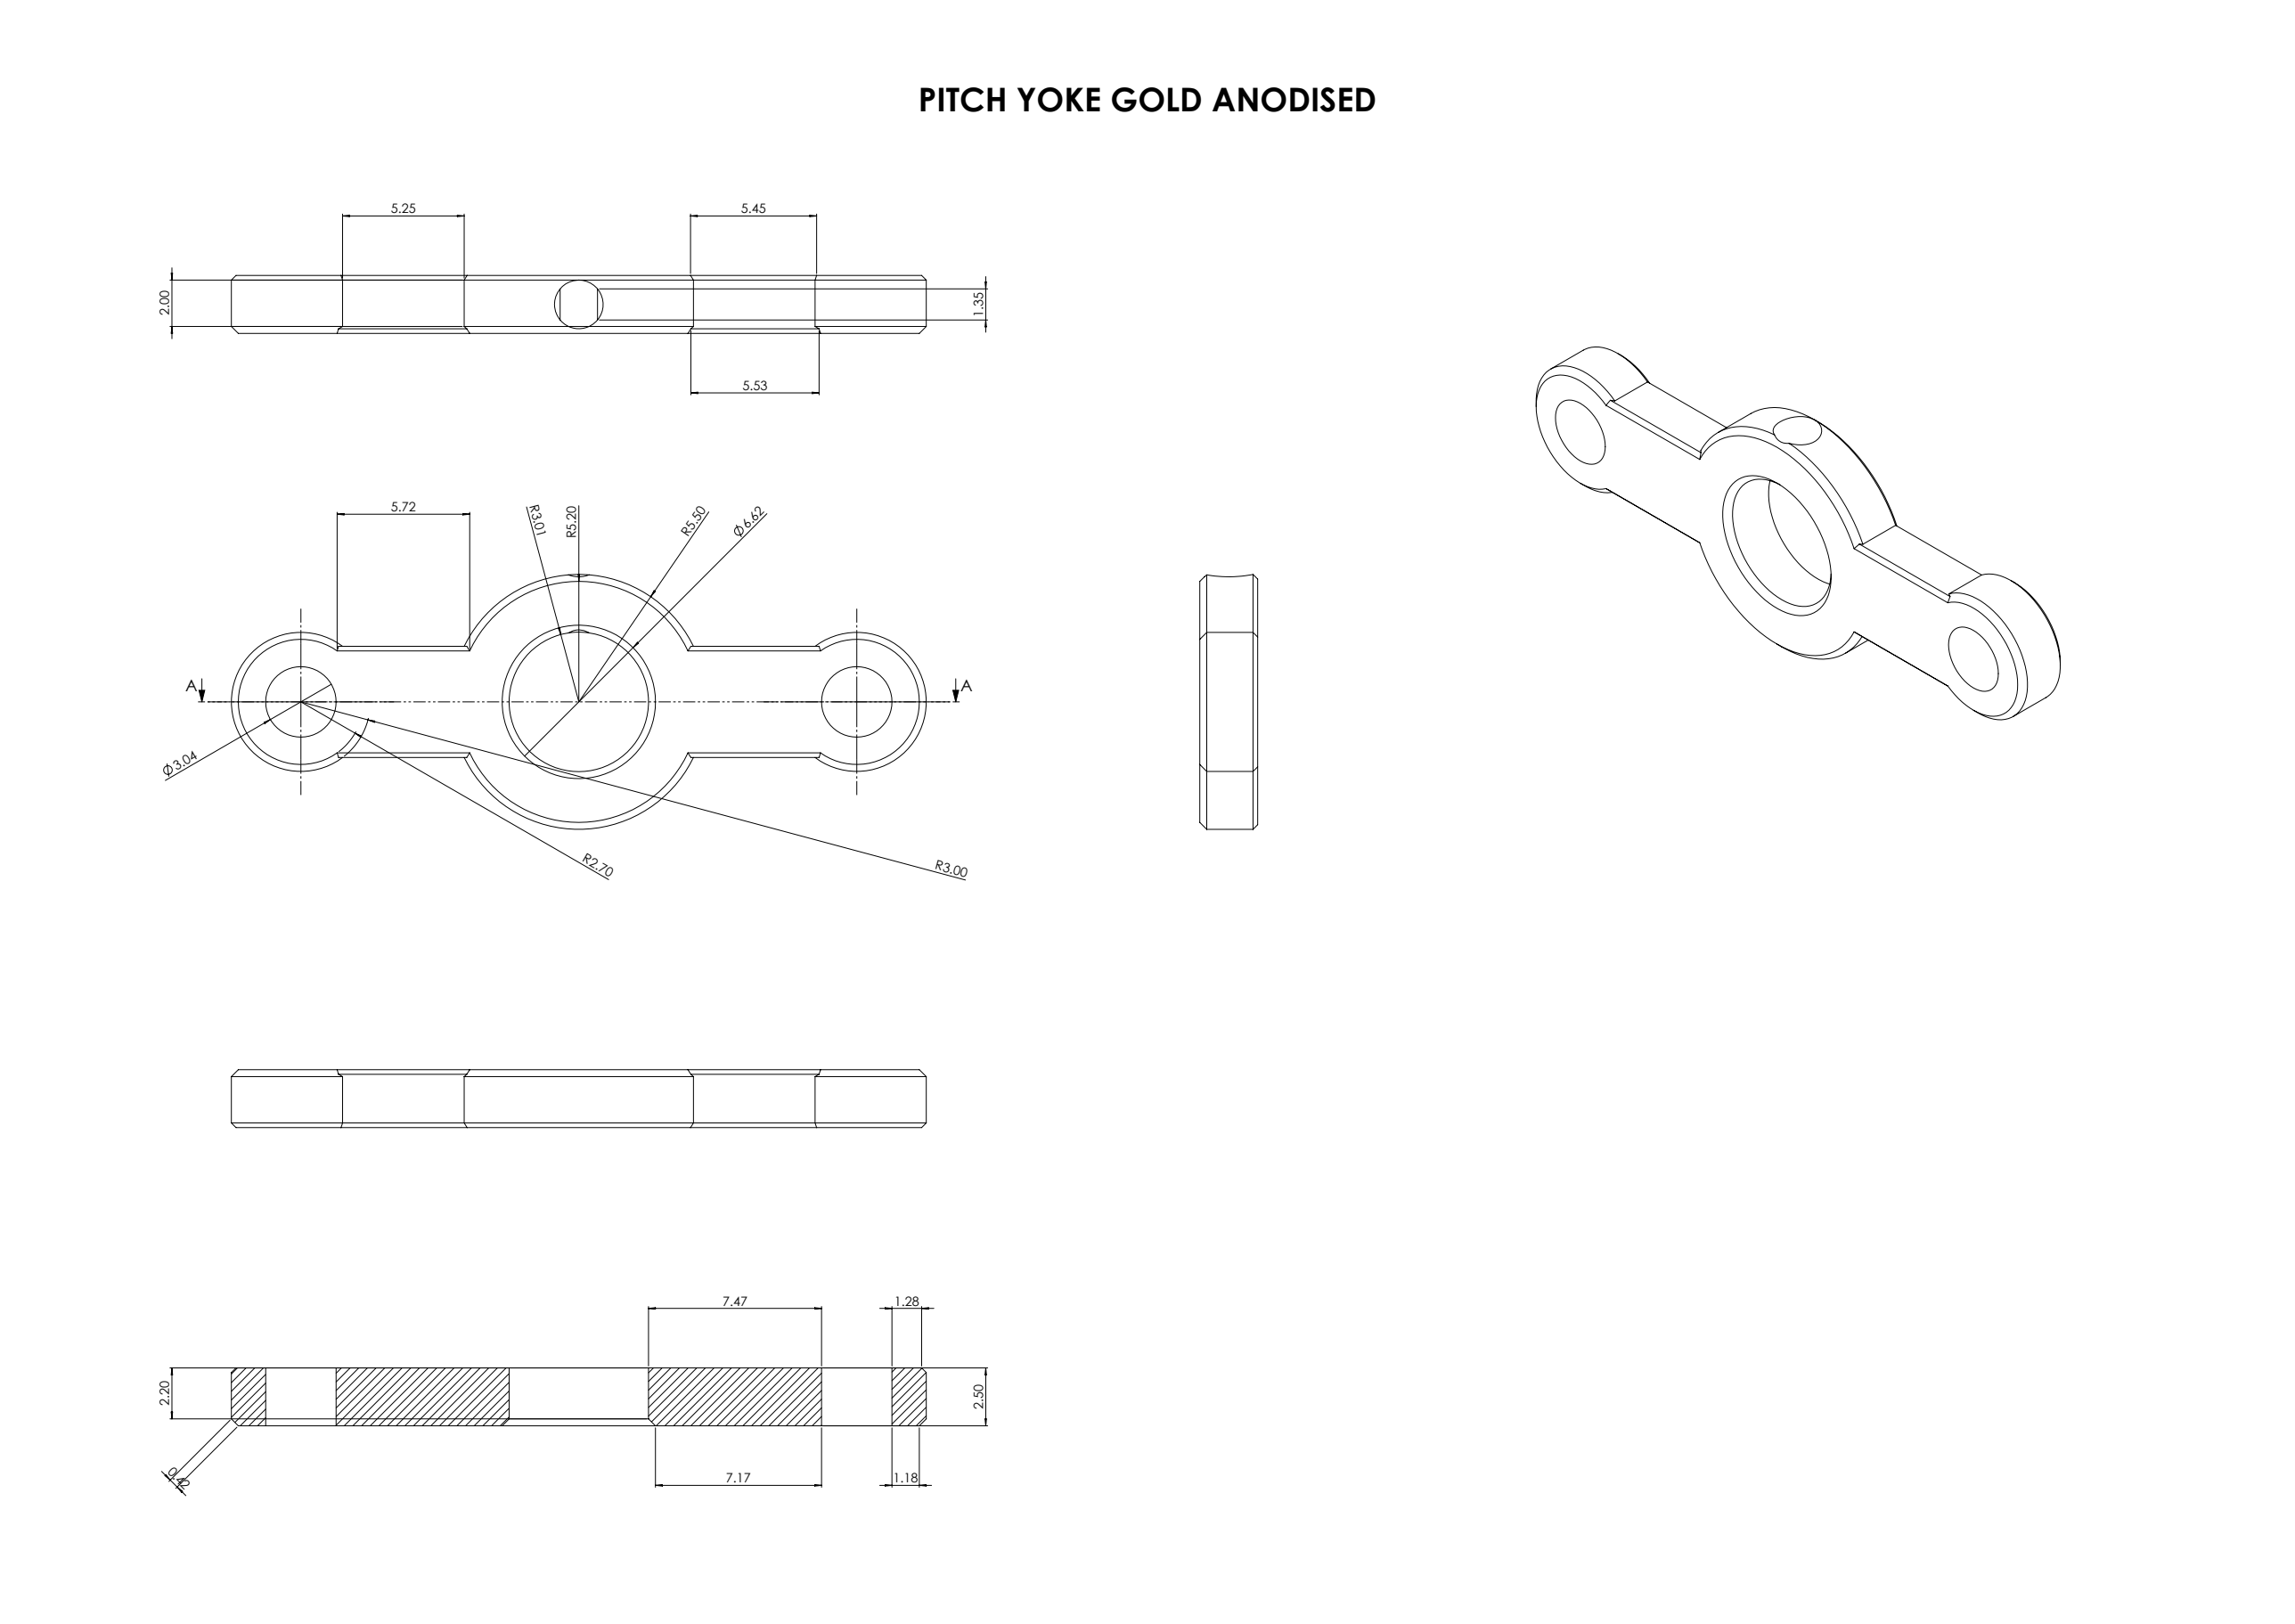
ISO-10303-21;
HEADER;
/* Generated by software containing ST-Developer
 * from STEP Tools, Inc. (www.steptools.com) 
 */

FILE_DESCRIPTION(
/* description */ (''),
/* implementation_level */ '2;1');

FILE_NAME(
/* name */ '05_Pitch_Yoke_Gold_Anodised.step',
/* time_stamp */ '2026-10-25T01:35:35-07:00',
/* author */ (''),
/* organization */ (''),
/* preprocessor_version */ 'ST-DEVELOPER v20.2',
/* originating_system */ 'Autodesk Translation Framework v15.15.0.0',
/* authorisation */ '');

FILE_SCHEMA (('AUTOMOTIVE_DESIGN { 1 0 10303 214 3 1 1 }'));
ENDSEC;

DATA;
#10=MECHANICAL_DESIGN_GEOMETRIC_PRESENTATION_REPRESENTATION('',(#264),#11430);
#86=B_SPLINE_CURVE_WITH_KNOTS('',3,(#6723,#6724,#6725,#6726),
 .UNSPECIFIED.,.F.,.F.,(4,4),(-0.0309968818258504,0.),.UNSPECIFIED.);
#87=B_SPLINE_CURVE_WITH_KNOTS('',3,(#6727,#6728,#6729,#6730),
 .UNSPECIFIED.,.F.,.F.,(4,4),(-0.0290771795561931,0.),.UNSPECIFIED.);
#88=B_SPLINE_CURVE_WITH_KNOTS('',3,(#6734,#6735,#6736,#6737),
 .UNSPECIFIED.,.F.,.F.,(4,4),(-0.0309968818257846,0.),.UNSPECIFIED.);
#89=B_SPLINE_CURVE_WITH_KNOTS('',3,(#6742,#6743,#6744,#6745),
 .UNSPECIFIED.,.F.,.F.,(4,4),(-0.0290773085804053,0.),.UNSPECIFIED.);
#90=B_SPLINE_CURVE_WITH_KNOTS('',3,(#6748,#6749,#6750,#6751),
 .UNSPECIFIED.,.F.,.F.,(4,4),(-0.0290771795561931,0.),.UNSPECIFIED.);
#91=B_SPLINE_CURVE_WITH_KNOTS('',3,(#6757,#6758,#6759,#6760),
 .UNSPECIFIED.,.F.,.F.,(4,4),(-0.0309968818258147,0.),.UNSPECIFIED.);
#92=B_SPLINE_CURVE_WITH_KNOTS('',3,(#6767,#6768,#6769,#6770),
 .UNSPECIFIED.,.F.,.F.,(4,4),(-0.030996881825835,0.),.UNSPECIFIED.);
#93=B_SPLINE_CURVE_WITH_KNOTS('',3,(#6774,#6775,#6776,#6777),
 .UNSPECIFIED.,.F.,.F.,(4,4),(-0.0290771795558996,0.),.UNSPECIFIED.);
#94=B_SPLINE_CURVE_WITH_KNOTS('',3,(#6787,#6788,#6789,#6790,#6791,#6792,
#6793,#6794,#6795,#6796,#6797,#6798,#6799,#6800,#6801,#6802,#6803),
 .UNSPECIFIED.,.F.,.F.,(4,2,2,2,3,2,2,4),(0.475883554626383,0.515539598201686,
0.555195641776989,0.594853523972749,0.63451140616851,0.674169288364271,
0.713827170560032,0.748840077704135),.UNSPECIFIED.);
#95=B_SPLINE_CURVE_WITH_KNOTS('',3,(#6818,#6819,#6820,#6821,#6822,#6823,
#6824,#6825,#6826,#6827),.UNSPECIFIED.,.F.,.F.,(4,2,2,2,4),(0.119476318069872,
0.130197921487587,0.164602551565189,0.199007181642792,0.209728785060507),
 .UNSPECIFIED.);
#96=B_SPLINE_CURVE_WITH_KNOTS('',3,(#6832,#6833,#6834,#6835,#6836,#6837,
#6838,#6839),.UNSPECIFIED.,.F.,.F.,(4,2,2,4),(0.20292703154863,0.237939938692733,
0.277597820888494,0.317255703084255),.UNSPECIFIED.);
#97=B_SPLINE_CURVE_WITH_KNOTS('',3,(#6840,#6841,#6842,#6843,#6844,#6845,
#6846,#6847,#6848,#6849),.UNSPECIFIED.,.F.,.F.,(4,2,2,2,4),(0.317255703084255,
0.356913585280016,0.396571467475777,0.43622751105108,0.475883554626383),
 .UNSPECIFIED.);
#98=B_SPLINE_CURVE_WITH_KNOTS('',3,(#6856,#6857,#6858,#6859,#6860,#6861,
#6862,#6863,#6864,#6865,#6866,#6867,#6868,#6869),.UNSPECIFIED.,.F.,.F.,
(4,2,2,2,2,2,4),(0.389725630667101,0.399201782687169,0.439108489087217,
0.479015195487264,0.518921901887312,0.55882860828736,0.568304760307428),
 .UNSPECIFIED.);
#99=B_SPLINE_CURVE_WITH_KNOTS('',3,(#6873,#6874,#6875,#6876,#6877,#6878),
 .UNSPECIFIED.,.F.,.F.,(4,2,4),(0.204141306797506,0.239485144629183,0.248961296649252),
 .UNSPECIFIED.);
#100=B_SPLINE_CURVE_WITH_KNOTS('',3,(#6880,#6881,#6882,#6883,#6884,#6885,
#6886,#6887,#6888,#6889),.UNSPECIFIED.,.F.,.F.,(4,2,2,2,4),(0.238592722720123,
0.259879734519813,0.28491657542964,0.309953416339467,0.331240428139157),
 .UNSPECIFIED.);
#101=B_SPLINE_CURVE_WITH_KNOTS('',3,(#6891,#6892,#6893,#6894,#6895,#6896),
 .UNSPECIFIED.,.F.,.F.,(4,2,4),(0.0703821670089247,0.079858319028993,0.115202156860671),
 .UNSPECIFIED.);
#220=(
BOUNDED_CURVE()
B_SPLINE_CURVE(2,(#6614,#6615,#6616),.UNSPECIFIED.,.F.,.F.)
B_SPLINE_CURVE_WITH_KNOTS((3,3),(0.,0.0309504086115576),.UNSPECIFIED.)
CURVE()
GEOMETRIC_REPRESENTATION_ITEM()
RATIONAL_B_SPLINE_CURVE((1.,1.,1.))
REPRESENTATION_ITEM('')
);
#221=(
BOUNDED_CURVE()
B_SPLINE_CURVE(2,(#6620,#6621,#6622),.UNSPECIFIED.,.F.,.F.)
B_SPLINE_CURVE_WITH_KNOTS((3,3),(0.,0.0289695421536074),.UNSPECIFIED.)
CURVE()
GEOMETRIC_REPRESENTATION_ITEM()
RATIONAL_B_SPLINE_CURVE((1.,1.,1.))
REPRESENTATION_ITEM('')
);
#222=(
BOUNDED_CURVE()
B_SPLINE_CURVE(2,(#6626,#6627,#6628),.UNSPECIFIED.,.F.,.F.)
B_SPLINE_CURVE_WITH_KNOTS((3,3),(0.0303639456287982,0.0450225821689597),
 .UNSPECIFIED.)
CURVE()
GEOMETRIC_REPRESENTATION_ITEM()
RATIONAL_B_SPLINE_CURVE((1.00021631089164,1.00016036906093,1.))
REPRESENTATION_ITEM('')
);
#223=(
BOUNDED_CURVE()
B_SPLINE_CURVE(2,(#6635,#6636,#6637),.UNSPECIFIED.,.F.,.F.)
B_SPLINE_CURVE_WITH_KNOTS((3,3),(0.,0.0187833832018332),.UNSPECIFIED.)
CURVE()
GEOMETRIC_REPRESENTATION_ITEM()
RATIONAL_B_SPLINE_CURVE((1.,1.0014465102333,1.00204161237231))
REPRESENTATION_ITEM('')
);
#224=(
BOUNDED_CURVE()
B_SPLINE_CURVE(2,(#6641,#6642,#6643),.UNSPECIFIED.,.F.,.F.)
B_SPLINE_CURVE_WITH_KNOTS((3,3),(0.,0.0289695421536071),.UNSPECIFIED.)
CURVE()
GEOMETRIC_REPRESENTATION_ITEM()
RATIONAL_B_SPLINE_CURVE((1.,1.,1.))
REPRESENTATION_ITEM('')
);
#225=(
BOUNDED_CURVE()
B_SPLINE_CURVE(2,(#6647,#6648,#6649),.UNSPECIFIED.,.F.,.F.)
B_SPLINE_CURVE_WITH_KNOTS((3,3),(0.,0.0309504086115573),.UNSPECIFIED.)
CURVE()
GEOMETRIC_REPRESENTATION_ITEM()
RATIONAL_B_SPLINE_CURVE((1.,1.,1.))
REPRESENTATION_ITEM('')
);
#226=(
BOUNDED_CURVE()
B_SPLINE_CURVE(2,(#6653,#6654,#6655),.UNSPECIFIED.,.F.,.F.)
B_SPLINE_CURVE_WITH_KNOTS((3,3),(0.0450411357331602,0.0638245189349933),
 .UNSPECIFIED.)
CURVE()
GEOMETRIC_REPRESENTATION_ITEM()
RATIONAL_B_SPLINE_CURVE((1.00204161237231,1.0014465102333,1.))
REPRESENTATION_ITEM('')
);
#227=(
BOUNDED_CURVE()
B_SPLINE_CURVE(2,(#6662,#6663,#6664),.UNSPECIFIED.,.F.,.F.)
B_SPLINE_CURVE_WITH_KNOTS((3,3),(0.,0.0146586365398684),.UNSPECIFIED.)
CURVE()
GEOMETRIC_REPRESENTATION_ITEM()
RATIONAL_B_SPLINE_CURVE((1.,1.00016036906092,1.00021631089164))
REPRESENTATION_ITEM('')
);
#228=(
BOUNDED_CURVE()
B_SPLINE_CURVE(2,(#6668,#6669,#6670),.UNSPECIFIED.,.F.,.F.)
B_SPLINE_CURVE_WITH_KNOTS((3,3),(0.,0.0309504086115573),.UNSPECIFIED.)
CURVE()
GEOMETRIC_REPRESENTATION_ITEM()
RATIONAL_B_SPLINE_CURVE((1.,1.,1.))
REPRESENTATION_ITEM('')
);
#229=(
BOUNDED_CURVE()
B_SPLINE_CURVE(2,(#6674,#6675,#6676),.UNSPECIFIED.,.F.,.F.)
B_SPLINE_CURVE_WITH_KNOTS((3,3),(0.,0.0289695421536071),.UNSPECIFIED.)
CURVE()
GEOMETRIC_REPRESENTATION_ITEM()
RATIONAL_B_SPLINE_CURVE((1.,1.,1.))
REPRESENTATION_ITEM('')
);
#230=(
BOUNDED_CURVE()
B_SPLINE_CURVE(2,(#6680,#6681,#6682),.UNSPECIFIED.,.F.,.F.)
B_SPLINE_CURVE_WITH_KNOTS((3,3),(0.0303678686581102,0.0450284286877096),
 .UNSPECIFIED.)
CURVE()
GEOMETRIC_REPRESENTATION_ITEM()
RATIONAL_B_SPLINE_CURVE((1.00021903389143,1.00016374915722,1.00000403669809))
REPRESENTATION_ITEM('')
);
#231=(
BOUNDED_CURVE()
B_SPLINE_CURVE(2,(#6689,#6690,#6691),.UNSPECIFIED.,.F.,.F.)
B_SPLINE_CURVE_WITH_KNOTS((3,3),(0.,0.0187833832018332),.UNSPECIFIED.)
CURVE()
GEOMETRIC_REPRESENTATION_ITEM()
RATIONAL_B_SPLINE_CURVE((1.,1.0014465102333,1.00204161237231))
REPRESENTATION_ITEM('')
);
#232=(
BOUNDED_CURVE()
B_SPLINE_CURVE(2,(#6695,#6696,#6697),.UNSPECIFIED.,.F.,.F.)
B_SPLINE_CURVE_WITH_KNOTS((3,3),(0.,0.0289695421536071),.UNSPECIFIED.)
CURVE()
GEOMETRIC_REPRESENTATION_ITEM()
RATIONAL_B_SPLINE_CURVE((1.,1.,1.))
REPRESENTATION_ITEM('')
);
#233=(
BOUNDED_CURVE()
B_SPLINE_CURVE(2,(#6701,#6702,#6703),.UNSPECIFIED.,.F.,.F.)
B_SPLINE_CURVE_WITH_KNOTS((3,3),(0.,0.0309504086115573),.UNSPECIFIED.)
CURVE()
GEOMETRIC_REPRESENTATION_ITEM()
RATIONAL_B_SPLINE_CURVE((1.,1.,1.))
REPRESENTATION_ITEM('')
);
#234=(
BOUNDED_CURVE()
B_SPLINE_CURVE(2,(#6707,#6708,#6709),.UNSPECIFIED.,.F.,.F.)
B_SPLINE_CURVE_WITH_KNOTS((3,3),(0.0450411357331602,0.0638245189349933),
 .UNSPECIFIED.)
CURVE()
GEOMETRIC_REPRESENTATION_ITEM()
RATIONAL_B_SPLINE_CURVE((1.00204161237231,1.0014465102333,1.))
REPRESENTATION_ITEM('')
);
#235=(
BOUNDED_CURVE()
B_SPLINE_CURVE(2,(#6716,#6717,#6718),.UNSPECIFIED.,.F.,.F.)
B_SPLINE_CURVE_WITH_KNOTS((3,3),(0.,0.014658636844145),.UNSPECIFIED.)
CURVE()
GEOMETRIC_REPRESENTATION_ITEM()
RATIONAL_B_SPLINE_CURVE((1.,1.00016036906825,1.00021631090007))
REPRESENTATION_ITEM('')
);
#240=SHAPE_REPRESENTATION_RELATIONSHIP('SRR','None',#11483,#252);
#252=ADVANCED_BREP_SHAPE_REPRESENTATION('',(#276),#11422);
#264=STYLED_ITEM('',(#11623),#276);
#276=MANIFOLD_SOLID_BREP('Body1',#4465);
#300=FACE_BOUND('',#901,.T.);
#301=FACE_BOUND('',#902,.T.);
#302=FACE_BOUND('',#903,.T.);
#303=FACE_BOUND('',#912,.T.);
#304=FACE_BOUND('',#913,.T.);
#305=FACE_BOUND('',#914,.T.);
#353=PLANE('',#4743);
#354=PLANE('',#4744);
#355=PLANE('',#4745);
#356=PLANE('',#4746);
#357=PLANE('',#4747);
#358=PLANE('',#4748);
#359=PLANE('',#4749);
#360=PLANE('',#4750);
#361=PLANE('',#4751);
#362=PLANE('',#4758);
#363=PLANE('',#4759);
#364=PLANE('',#4764);
#365=PLANE('',#4776);
#366=PLANE('',#4798);
#367=PLANE('',#4801);
#368=PLANE('',#4802);
#447=CYLINDRICAL_SURFACE('',#4768,3.);
#448=CYLINDRICAL_SURFACE('',#4770,5.5);
#449=CYLINDRICAL_SURFACE('',#4772,5.5);
#450=CYLINDRICAL_SURFACE('',#4774,3.);
#451=CYLINDRICAL_SURFACE('',#4785,5.5);
#452=CYLINDRICAL_SURFACE('',#4786,1.05);
#453=CYLINDRICAL_SURFACE('',#4803,1.52);
#454=CYLINDRICAL_SURFACE('',#4804,1.52);
#455=CYLINDRICAL_SURFACE('',#4805,3.01);
#596=FACE_OUTER_BOUND('',#880,.T.);
#597=FACE_OUTER_BOUND('',#881,.T.);
#598=FACE_OUTER_BOUND('',#882,.T.);
#599=FACE_OUTER_BOUND('',#883,.T.);
#600=FACE_OUTER_BOUND('',#884,.T.);
#601=FACE_OUTER_BOUND('',#885,.T.);
#602=FACE_OUTER_BOUND('',#886,.T.);
#603=FACE_OUTER_BOUND('',#887,.T.);
#604=FACE_OUTER_BOUND('',#888,.T.);
#605=FACE_OUTER_BOUND('',#889,.T.);
#606=FACE_OUTER_BOUND('',#890,.T.);
#607=FACE_OUTER_BOUND('',#891,.T.);
#608=FACE_OUTER_BOUND('',#892,.T.);
#609=FACE_OUTER_BOUND('',#893,.T.);
#610=FACE_OUTER_BOUND('',#894,.T.);
#611=FACE_OUTER_BOUND('',#895,.T.);
#612=FACE_OUTER_BOUND('',#896,.T.);
#613=FACE_OUTER_BOUND('',#897,.T.);
#614=FACE_OUTER_BOUND('',#898,.T.);
#615=FACE_OUTER_BOUND('',#899,.T.);
#616=FACE_OUTER_BOUND('',#900,.T.);
#617=FACE_OUTER_BOUND('',#904,.T.);
#618=FACE_OUTER_BOUND('',#905,.T.);
#619=FACE_OUTER_BOUND('',#906,.T.);
#620=FACE_OUTER_BOUND('',#907,.T.);
#621=FACE_OUTER_BOUND('',#908,.T.);
#622=FACE_OUTER_BOUND('',#909,.T.);
#623=FACE_OUTER_BOUND('',#910,.T.);
#624=FACE_OUTER_BOUND('',#911,.T.);
#625=FACE_OUTER_BOUND('',#915,.T.);
#626=FACE_OUTER_BOUND('',#916,.T.);
#627=FACE_OUTER_BOUND('',#917,.T.);
#628=FACE_OUTER_BOUND('',#918,.T.);
#629=FACE_OUTER_BOUND('',#919,.T.);
#880=EDGE_LOOP('',(#3147,#3148,#3149,#3150));
#881=EDGE_LOOP('',(#3151,#3152,#3153,#3154,#3155,#3156));
#882=EDGE_LOOP('',(#3157,#3158,#3159,#3160));
#883=EDGE_LOOP('',(#3161,#3162,#3163,#3164,#3165,#3166));
#884=EDGE_LOOP('',(#3167,#3168,#3169,#3170));
#885=EDGE_LOOP('',(#3171,#3172,#3173,#3174,#3175,#3176));
#886=EDGE_LOOP('',(#3177,#3178,#3179,#3180));
#887=EDGE_LOOP('',(#3181,#3182,#3183,#3184,#3185,#3186));
#888=EDGE_LOOP('',(#3187,#3188,#3189,#3190));
#889=EDGE_LOOP('',(#3191,#3192,#3193,#3194));
#890=EDGE_LOOP('',(#3195,#3196,#3197,#3198));
#891=EDGE_LOOP('',(#3199,#3200,#3201,#3202));
#892=EDGE_LOOP('',(#3203,#3204,#3205,#3206));
#893=EDGE_LOOP('',(#3207,#3208,#3209,#3210,#3211));
#894=EDGE_LOOP('',(#3212,#3213,#3214,#3215));
#895=EDGE_LOOP('',(#3216,#3217,#3218,#3219));
#896=EDGE_LOOP('',(#3220,#3221,#3222,#3223));
#897=EDGE_LOOP('',(#3224,#3225,#3226,#3227));
#898=EDGE_LOOP('',(#3228,#3229,#3230,#3231));
#899=EDGE_LOOP('',(#3232,#3233,#3234,#3235));
#900=EDGE_LOOP('',(#3236,#3237,#3238,#3239,#3240,#3241,#3242,#3243));
#901=EDGE_LOOP('',(#3244));
#902=EDGE_LOOP('',(#3245));
#903=EDGE_LOOP('',(#3246));
#904=EDGE_LOOP('',(#3247,#3248,#3249,#3250,#3251,#3252));
#905=EDGE_LOOP('',(#3253,#3254,#3255,#3256,#3257,#3258,#3259,#3260));
#906=EDGE_LOOP('',(#3261,#3262,#3263,#3264,#3265));
#907=EDGE_LOOP('',(#3266,#3267,#3268,#3269,#3270,#3271,#3272,#3273,#3274,
#3275,#3276,#3277,#3278));
#908=EDGE_LOOP('',(#3279,#3280,#3281,#3282,#3283,#3284));
#909=EDGE_LOOP('',(#3285,#3286,#3287,#3288,#3289,#3290));
#910=EDGE_LOOP('',(#3291,#3292,#3293,#3294,#3295,#3296));
#911=EDGE_LOOP('',(#3297,#3298,#3299,#3300,#3301,#3302,#3303,#3304));
#912=EDGE_LOOP('',(#3305));
#913=EDGE_LOOP('',(#3306));
#914=EDGE_LOOP('',(#3307));
#915=EDGE_LOOP('',(#3308,#3309,#3310));
#916=EDGE_LOOP('',(#3311,#3312));
#917=EDGE_LOOP('',(#3313,#3314,#3315,#3316));
#918=EDGE_LOOP('',(#3317,#3318,#3319,#3320));
#919=EDGE_LOOP('',(#3321,#3322,#3323,#3324,#3325,#3326,#3327,#3328,#3329,
#3330));
#1171=LINE('',#6618,#1461);
#1172=LINE('',#6623,#1462);
#1173=LINE('',#6630,#1463);
#1174=LINE('',#6632,#1464);
#1175=LINE('',#6634,#1465);
#1176=LINE('',#6645,#1466);
#1177=LINE('',#6650,#1467);
#1178=LINE('',#6657,#1468);
#1179=LINE('',#6659,#1469);
#1180=LINE('',#6661,#1470);
#1181=LINE('',#6672,#1471);
#1182=LINE('',#6677,#1472);
#1183=LINE('',#6684,#1473);
#1184=LINE('',#6686,#1474);
#1185=LINE('',#6688,#1475);
#1186=LINE('',#6699,#1476);
#1187=LINE('',#6704,#1477);
#1188=LINE('',#6711,#1478);
#1189=LINE('',#6713,#1479);
#1190=LINE('',#6715,#1480);
#1191=LINE('',#6722,#1481);
#1192=LINE('',#6753,#1482);
#1193=LINE('',#6756,#1483);
#1194=LINE('',#6773,#1484);
#1195=LINE('',#6852,#1485);
#1196=LINE('',#6906,#1486);
#1197=LINE('',#6915,#1487);
#1198=LINE('',#6917,#1488);
#1199=LINE('',#6919,#1489);
#1200=LINE('',#6921,#1490);
#1201=LINE('',#6923,#1491);
#1461=VECTOR('',#5429,10.);
#1462=VECTOR('',#5430,10.);
#1463=VECTOR('',#5433,10.);
#1464=VECTOR('',#5434,10.);
#1465=VECTOR('',#5435,10.);
#1466=VECTOR('',#5438,10.);
#1467=VECTOR('',#5439,10.);
#1468=VECTOR('',#5442,10.);
#1469=VECTOR('',#5443,10.);
#1470=VECTOR('',#5444,10.);
#1471=VECTOR('',#5447,10.);
#1472=VECTOR('',#5448,10.);
#1473=VECTOR('',#5451,10.);
#1474=VECTOR('',#5452,10.);
#1475=VECTOR('',#5453,10.);
#1476=VECTOR('',#5456,10.);
#1477=VECTOR('',#5457,10.);
#1478=VECTOR('',#5460,10.);
#1479=VECTOR('',#5461,10.);
#1480=VECTOR('',#5462,10.);
#1481=VECTOR('',#5465,10.);
#1482=VECTOR('',#5480,10.);
#1483=VECTOR('',#5483,10.);
#1484=VECTOR('',#5494,10.);
#1485=VECTOR('',#5539,1.05);
#1486=VECTOR('',#5558,3.16);
#1487=VECTOR('',#5571,10.);
#1488=VECTOR('',#5574,10.);
#1489=VECTOR('',#5577,1.52);
#1490=VECTOR('',#5580,1.52);
#1491=VECTOR('',#5583,3.01);
#1742=CIRCLE('',#4753,5.3);
#1743=CIRCLE('',#4754,5.5);
#1744=CIRCLE('',#4756,3.);
#1745=CIRCLE('',#4757,2.8);
#1746=CIRCLE('',#4761,5.5);
#1747=CIRCLE('',#4762,5.5);
#1748=CIRCLE('',#4763,5.3);
#1749=CIRCLE('',#4766,3.);
#1750=CIRCLE('',#4767,2.8);
#1751=CIRCLE('',#4769,3.);
#1752=CIRCLE('',#4771,5.5);
#1753=CIRCLE('',#4773,5.5);
#1754=CIRCLE('',#4775,3.);
#1755=CIRCLE('',#4777,3.01);
#1756=CIRCLE('',#4778,1.52);
#1757=CIRCLE('',#4779,1.52);
#1758=CIRCLE('',#4781,2.7);
#1759=CIRCLE('',#4783,5.5);
#1760=CIRCLE('',#4784,5.2);
#1761=CIRCLE('',#4787,1.05);
#1762=CIRCLE('',#4788,1.05);
#1763=CIRCLE('',#4789,1.05);
#1764=CIRCLE('',#4791,2.7);
#1765=CIRCLE('',#4793,5.2);
#1766=CIRCLE('',#4795,3.31);
#1767=CIRCLE('',#4796,3.01);
#1768=CIRCLE('',#4797,3.01);
#1769=CIRCLE('',#4799,1.52);
#1770=CIRCLE('',#4800,1.52);
#1943=VERTEX_POINT('',#6612);
#1944=VERTEX_POINT('',#6613);
#1945=VERTEX_POINT('',#6617);
#1946=VERTEX_POINT('',#6619);
#1947=VERTEX_POINT('',#6625);
#1948=VERTEX_POINT('',#6629);
#1949=VERTEX_POINT('',#6631);
#1950=VERTEX_POINT('',#6633);
#1951=VERTEX_POINT('',#6639);
#1952=VERTEX_POINT('',#6640);
#1953=VERTEX_POINT('',#6644);
#1954=VERTEX_POINT('',#6646);
#1955=VERTEX_POINT('',#6652);
#1956=VERTEX_POINT('',#6656);
#1957=VERTEX_POINT('',#6658);
#1958=VERTEX_POINT('',#6660);
#1959=VERTEX_POINT('',#6666);
#1960=VERTEX_POINT('',#6667);
#1961=VERTEX_POINT('',#6671);
#1962=VERTEX_POINT('',#6673);
#1963=VERTEX_POINT('',#6679);
#1964=VERTEX_POINT('',#6683);
#1965=VERTEX_POINT('',#6685);
#1966=VERTEX_POINT('',#6687);
#1967=VERTEX_POINT('',#6693);
#1968=VERTEX_POINT('',#6694);
#1969=VERTEX_POINT('',#6698);
#1970=VERTEX_POINT('',#6700);
#1971=VERTEX_POINT('',#6706);
#1972=VERTEX_POINT('',#6710);
#1973=VERTEX_POINT('',#6712);
#1974=VERTEX_POINT('',#6714);
#1975=VERTEX_POINT('',#6720);
#1976=VERTEX_POINT('',#6721);
#1977=VERTEX_POINT('',#6732);
#1978=VERTEX_POINT('',#6741);
#1979=VERTEX_POINT('',#6746);
#1980=VERTEX_POINT('',#6755);
#1981=VERTEX_POINT('',#6762);
#1982=VERTEX_POINT('',#6765);
#1983=VERTEX_POINT('',#6772);
#1984=VERTEX_POINT('',#6786);
#1985=VERTEX_POINT('',#6808);
#1986=VERTEX_POINT('',#6810);
#1987=VERTEX_POINT('',#6812);
#1988=VERTEX_POINT('',#6817);
#1989=VERTEX_POINT('',#6831);
#1990=VERTEX_POINT('',#6851);
#1991=VERTEX_POINT('',#6853);
#1992=VERTEX_POINT('',#6855);
#1993=VERTEX_POINT('',#6870);
#1994=VERTEX_POINT('',#6872);
#1995=VERTEX_POINT('',#6879);
#1996=VERTEX_POINT('',#6890);
#1997=VERTEX_POINT('',#6903);
#1998=VERTEX_POINT('',#6905);
#1999=VERTEX_POINT('',#6910);
#2000=VERTEX_POINT('',#6912);
#2391=EDGE_CURVE('',#1943,#1944,#220,.F.);
#2392=EDGE_CURVE('',#1944,#1945,#1171,.T.);
#2393=EDGE_CURVE('',#1945,#1946,#221,.F.);
#2394=EDGE_CURVE('',#1946,#1943,#1172,.T.);
#2395=EDGE_CURVE('',#1947,#1944,#222,.F.);
#2396=EDGE_CURVE('',#1948,#1947,#1173,.T.);
#2397=EDGE_CURVE('',#1949,#1948,#1174,.T.);
#2398=EDGE_CURVE('',#1949,#1950,#1175,.T.);
#2399=EDGE_CURVE('',#1945,#1950,#223,.F.);
#2400=EDGE_CURVE('',#1951,#1952,#224,.F.);
#2401=EDGE_CURVE('',#1952,#1953,#1176,.T.);
#2402=EDGE_CURVE('',#1953,#1954,#225,.F.);
#2403=EDGE_CURVE('',#1954,#1951,#1177,.T.);
#2404=EDGE_CURVE('',#1955,#1952,#226,.F.);
#2405=EDGE_CURVE('',#1956,#1955,#1178,.T.);
#2406=EDGE_CURVE('',#1957,#1956,#1179,.T.);
#2407=EDGE_CURVE('',#1957,#1958,#1180,.T.);
#2408=EDGE_CURVE('',#1953,#1958,#227,.F.);
#2409=EDGE_CURVE('',#1959,#1960,#228,.F.);
#2410=EDGE_CURVE('',#1960,#1961,#1181,.T.);
#2411=EDGE_CURVE('',#1961,#1962,#229,.F.);
#2412=EDGE_CURVE('',#1962,#1959,#1182,.T.);
#2413=EDGE_CURVE('',#1963,#1960,#230,.F.);
#2414=EDGE_CURVE('',#1964,#1963,#1183,.T.);
#2415=EDGE_CURVE('',#1965,#1964,#1184,.T.);
#2416=EDGE_CURVE('',#1965,#1966,#1185,.T.);
#2417=EDGE_CURVE('',#1961,#1966,#231,.F.);
#2418=EDGE_CURVE('',#1967,#1968,#232,.F.);
#2419=EDGE_CURVE('',#1968,#1969,#1186,.T.);
#2420=EDGE_CURVE('',#1969,#1970,#233,.F.);
#2421=EDGE_CURVE('',#1970,#1967,#1187,.T.);
#2422=EDGE_CURVE('',#1971,#1968,#234,.F.);
#2423=EDGE_CURVE('',#1972,#1971,#1188,.T.);
#2424=EDGE_CURVE('',#1973,#1972,#1189,.T.);
#2425=EDGE_CURVE('',#1973,#1974,#1190,.T.);
#2426=EDGE_CURVE('',#1969,#1974,#235,.F.);
#2427=EDGE_CURVE('',#1975,#1976,#1191,.T.);
#2428=EDGE_CURVE('',#1976,#1957,#86,.T.);
#2429=EDGE_CURVE('',#1975,#1956,#87,.T.);
#2430=EDGE_CURVE('',#1976,#1977,#1742,.T.);
#2431=EDGE_CURVE('',#1977,#1948,#88,.T.);
#2432=EDGE_CURVE('',#1948,#1957,#1743,.T.);
#2433=EDGE_CURVE('',#1972,#1949,#1744,.T.);
#2434=EDGE_CURVE('',#1949,#1978,#89,.T.);
#2435=EDGE_CURVE('',#1978,#1979,#1745,.T.);
#2436=EDGE_CURVE('',#1979,#1972,#90,.T.);
#2437=EDGE_CURVE('',#1977,#1978,#1192,.T.);
#2438=EDGE_CURVE('',#1979,#1980,#1193,.T.);
#2439=EDGE_CURVE('',#1980,#1973,#91,.T.);
#2440=EDGE_CURVE('',#1964,#1981,#1746,.T.);
#2441=EDGE_CURVE('',#1981,#1973,#1747,.T.);
#2442=EDGE_CURVE('',#1980,#1982,#1748,.T.);
#2443=EDGE_CURVE('',#1982,#1964,#92,.T.);
#2444=EDGE_CURVE('',#1982,#1983,#1194,.T.);
#2445=EDGE_CURVE('',#1983,#1965,#93,.T.);
#2446=EDGE_CURVE('',#1956,#1965,#1749,.T.);
#2447=EDGE_CURVE('',#1983,#1975,#1750,.T.);
#2448=EDGE_CURVE('',#1966,#1955,#1751,.T.);
#2449=EDGE_CURVE('',#1958,#1947,#1752,.T.);
#2450=EDGE_CURVE('',#1981,#1984,#94,.T.);
#2451=EDGE_CURVE('',#1974,#1984,#1753,.T.);
#2452=EDGE_CURVE('',#1950,#1971,#1754,.T.);
#2453=EDGE_CURVE('',#1985,#1985,#1755,.T.);
#2454=EDGE_CURVE('',#1986,#1986,#1756,.T.);
#2455=EDGE_CURVE('',#1987,#1987,#1757,.T.);
#2456=EDGE_CURVE('',#1967,#1946,#1758,.T.);
#2457=EDGE_CURVE('',#1984,#1988,#95,.T.);
#2458=EDGE_CURVE('',#1988,#1963,#1759,.T.);
#2459=EDGE_CURVE('',#1959,#1970,#1760,.T.);
#2460=EDGE_CURVE('',#1988,#1989,#96,.T.);
#2461=EDGE_CURVE('',#1989,#1981,#97,.T.);
#2462=EDGE_CURVE('',#1989,#1990,#1195,.T.);
#2463=EDGE_CURVE('',#1990,#1991,#1761,.T.);
#2464=EDGE_CURVE('',#1992,#1991,#98,.T.);
#2465=EDGE_CURVE('',#1992,#1993,#1762,.T.);
#2466=EDGE_CURVE('',#1994,#1993,#99,.T.);
#2467=EDGE_CURVE('',#1995,#1994,#100,.T.);
#2468=EDGE_CURVE('',#1996,#1995,#101,.T.);
#2469=EDGE_CURVE('',#1996,#1990,#1763,.T.);
#2470=EDGE_CURVE('',#1951,#1962,#1764,.T.);
#2471=EDGE_CURVE('',#1943,#1954,#1765,.T.);
#2472=EDGE_CURVE('',#1997,#1997,#1766,.T.);
#2473=EDGE_CURVE('',#1997,#1998,#1196,.T.);
#2474=EDGE_CURVE('',#1998,#1995,#1767,.T.);
#2475=EDGE_CURVE('',#1994,#1998,#1768,.T.);
#2476=EDGE_CURVE('',#1999,#1999,#1769,.T.);
#2477=EDGE_CURVE('',#2000,#2000,#1770,.T.);
#2478=EDGE_CURVE('',#1991,#1996,#1197,.T.);
#2479=EDGE_CURVE('',#1993,#1992,#1198,.T.);
#2480=EDGE_CURVE('',#2000,#1987,#1199,.T.);
#2481=EDGE_CURVE('',#1999,#1986,#1200,.T.);
#2482=EDGE_CURVE('',#1998,#1985,#1201,.T.);
#3147=ORIENTED_EDGE('',*,*,#2391,.T.);
#3148=ORIENTED_EDGE('',*,*,#2392,.T.);
#3149=ORIENTED_EDGE('',*,*,#2393,.T.);
#3150=ORIENTED_EDGE('',*,*,#2394,.T.);
#3151=ORIENTED_EDGE('',*,*,#2392,.F.);
#3152=ORIENTED_EDGE('',*,*,#2395,.F.);
#3153=ORIENTED_EDGE('',*,*,#2396,.F.);
#3154=ORIENTED_EDGE('',*,*,#2397,.F.);
#3155=ORIENTED_EDGE('',*,*,#2398,.T.);
#3156=ORIENTED_EDGE('',*,*,#2399,.F.);
#3157=ORIENTED_EDGE('',*,*,#2400,.T.);
#3158=ORIENTED_EDGE('',*,*,#2401,.T.);
#3159=ORIENTED_EDGE('',*,*,#2402,.T.);
#3160=ORIENTED_EDGE('',*,*,#2403,.T.);
#3161=ORIENTED_EDGE('',*,*,#2401,.F.);
#3162=ORIENTED_EDGE('',*,*,#2404,.F.);
#3163=ORIENTED_EDGE('',*,*,#2405,.F.);
#3164=ORIENTED_EDGE('',*,*,#2406,.F.);
#3165=ORIENTED_EDGE('',*,*,#2407,.T.);
#3166=ORIENTED_EDGE('',*,*,#2408,.F.);
#3167=ORIENTED_EDGE('',*,*,#2409,.T.);
#3168=ORIENTED_EDGE('',*,*,#2410,.T.);
#3169=ORIENTED_EDGE('',*,*,#2411,.T.);
#3170=ORIENTED_EDGE('',*,*,#2412,.T.);
#3171=ORIENTED_EDGE('',*,*,#2410,.F.);
#3172=ORIENTED_EDGE('',*,*,#2413,.F.);
#3173=ORIENTED_EDGE('',*,*,#2414,.F.);
#3174=ORIENTED_EDGE('',*,*,#2415,.F.);
#3175=ORIENTED_EDGE('',*,*,#2416,.T.);
#3176=ORIENTED_EDGE('',*,*,#2417,.F.);
#3177=ORIENTED_EDGE('',*,*,#2418,.T.);
#3178=ORIENTED_EDGE('',*,*,#2419,.T.);
#3179=ORIENTED_EDGE('',*,*,#2420,.T.);
#3180=ORIENTED_EDGE('',*,*,#2421,.T.);
#3181=ORIENTED_EDGE('',*,*,#2419,.F.);
#3182=ORIENTED_EDGE('',*,*,#2422,.F.);
#3183=ORIENTED_EDGE('',*,*,#2423,.F.);
#3184=ORIENTED_EDGE('',*,*,#2424,.F.);
#3185=ORIENTED_EDGE('',*,*,#2425,.T.);
#3186=ORIENTED_EDGE('',*,*,#2426,.F.);
#3187=ORIENTED_EDGE('',*,*,#2427,.T.);
#3188=ORIENTED_EDGE('',*,*,#2428,.T.);
#3189=ORIENTED_EDGE('',*,*,#2406,.T.);
#3190=ORIENTED_EDGE('',*,*,#2429,.F.);
#3191=ORIENTED_EDGE('',*,*,#2430,.T.);
#3192=ORIENTED_EDGE('',*,*,#2431,.T.);
#3193=ORIENTED_EDGE('',*,*,#2432,.T.);
#3194=ORIENTED_EDGE('',*,*,#2428,.F.);
#3195=ORIENTED_EDGE('',*,*,#2433,.T.);
#3196=ORIENTED_EDGE('',*,*,#2434,.T.);
#3197=ORIENTED_EDGE('',*,*,#2435,.T.);
#3198=ORIENTED_EDGE('',*,*,#2436,.T.);
#3199=ORIENTED_EDGE('',*,*,#2437,.T.);
#3200=ORIENTED_EDGE('',*,*,#2434,.F.);
#3201=ORIENTED_EDGE('',*,*,#2397,.T.);
#3202=ORIENTED_EDGE('',*,*,#2431,.F.);
#3203=ORIENTED_EDGE('',*,*,#2424,.T.);
#3204=ORIENTED_EDGE('',*,*,#2436,.F.);
#3205=ORIENTED_EDGE('',*,*,#2438,.T.);
#3206=ORIENTED_EDGE('',*,*,#2439,.T.);
#3207=ORIENTED_EDGE('',*,*,#2440,.T.);
#3208=ORIENTED_EDGE('',*,*,#2441,.T.);
#3209=ORIENTED_EDGE('',*,*,#2439,.F.);
#3210=ORIENTED_EDGE('',*,*,#2442,.T.);
#3211=ORIENTED_EDGE('',*,*,#2443,.T.);
#3212=ORIENTED_EDGE('',*,*,#2415,.T.);
#3213=ORIENTED_EDGE('',*,*,#2443,.F.);
#3214=ORIENTED_EDGE('',*,*,#2444,.T.);
#3215=ORIENTED_EDGE('',*,*,#2445,.T.);
#3216=ORIENTED_EDGE('',*,*,#2446,.T.);
#3217=ORIENTED_EDGE('',*,*,#2445,.F.);
#3218=ORIENTED_EDGE('',*,*,#2447,.T.);
#3219=ORIENTED_EDGE('',*,*,#2429,.T.);
#3220=ORIENTED_EDGE('',*,*,#2446,.F.);
#3221=ORIENTED_EDGE('',*,*,#2405,.T.);
#3222=ORIENTED_EDGE('',*,*,#2448,.F.);
#3223=ORIENTED_EDGE('',*,*,#2416,.F.);
#3224=ORIENTED_EDGE('',*,*,#2432,.F.);
#3225=ORIENTED_EDGE('',*,*,#2396,.T.);
#3226=ORIENTED_EDGE('',*,*,#2449,.F.);
#3227=ORIENTED_EDGE('',*,*,#2407,.F.);
#3228=ORIENTED_EDGE('',*,*,#2441,.F.);
#3229=ORIENTED_EDGE('',*,*,#2450,.T.);
#3230=ORIENTED_EDGE('',*,*,#2451,.F.);
#3231=ORIENTED_EDGE('',*,*,#2425,.F.);
#3232=ORIENTED_EDGE('',*,*,#2433,.F.);
#3233=ORIENTED_EDGE('',*,*,#2423,.T.);
#3234=ORIENTED_EDGE('',*,*,#2452,.F.);
#3235=ORIENTED_EDGE('',*,*,#2398,.F.);
#3236=ORIENTED_EDGE('',*,*,#2435,.F.);
#3237=ORIENTED_EDGE('',*,*,#2437,.F.);
#3238=ORIENTED_EDGE('',*,*,#2430,.F.);
#3239=ORIENTED_EDGE('',*,*,#2427,.F.);
#3240=ORIENTED_EDGE('',*,*,#2447,.F.);
#3241=ORIENTED_EDGE('',*,*,#2444,.F.);
#3242=ORIENTED_EDGE('',*,*,#2442,.F.);
#3243=ORIENTED_EDGE('',*,*,#2438,.F.);
#3244=ORIENTED_EDGE('',*,*,#2453,.T.);
#3245=ORIENTED_EDGE('',*,*,#2454,.T.);
#3246=ORIENTED_EDGE('',*,*,#2455,.T.);
#3247=ORIENTED_EDGE('',*,*,#2399,.T.);
#3248=ORIENTED_EDGE('',*,*,#2452,.T.);
#3249=ORIENTED_EDGE('',*,*,#2422,.T.);
#3250=ORIENTED_EDGE('',*,*,#2418,.F.);
#3251=ORIENTED_EDGE('',*,*,#2456,.T.);
#3252=ORIENTED_EDGE('',*,*,#2393,.F.);
#3253=ORIENTED_EDGE('',*,*,#2457,.T.);
#3254=ORIENTED_EDGE('',*,*,#2458,.T.);
#3255=ORIENTED_EDGE('',*,*,#2413,.T.);
#3256=ORIENTED_EDGE('',*,*,#2409,.F.);
#3257=ORIENTED_EDGE('',*,*,#2459,.T.);
#3258=ORIENTED_EDGE('',*,*,#2420,.F.);
#3259=ORIENTED_EDGE('',*,*,#2426,.T.);
#3260=ORIENTED_EDGE('',*,*,#2451,.T.);
#3261=ORIENTED_EDGE('',*,*,#2440,.F.);
#3262=ORIENTED_EDGE('',*,*,#2414,.T.);
#3263=ORIENTED_EDGE('',*,*,#2458,.F.);
#3264=ORIENTED_EDGE('',*,*,#2460,.T.);
#3265=ORIENTED_EDGE('',*,*,#2461,.T.);
#3266=ORIENTED_EDGE('',*,*,#2457,.F.);
#3267=ORIENTED_EDGE('',*,*,#2450,.F.);
#3268=ORIENTED_EDGE('',*,*,#2461,.F.);
#3269=ORIENTED_EDGE('',*,*,#2462,.T.);
#3270=ORIENTED_EDGE('',*,*,#2463,.T.);
#3271=ORIENTED_EDGE('',*,*,#2464,.F.);
#3272=ORIENTED_EDGE('',*,*,#2465,.T.);
#3273=ORIENTED_EDGE('',*,*,#2466,.F.);
#3274=ORIENTED_EDGE('',*,*,#2467,.F.);
#3275=ORIENTED_EDGE('',*,*,#2468,.F.);
#3276=ORIENTED_EDGE('',*,*,#2469,.T.);
#3277=ORIENTED_EDGE('',*,*,#2462,.F.);
#3278=ORIENTED_EDGE('',*,*,#2460,.F.);
#3279=ORIENTED_EDGE('',*,*,#2417,.T.);
#3280=ORIENTED_EDGE('',*,*,#2448,.T.);
#3281=ORIENTED_EDGE('',*,*,#2404,.T.);
#3282=ORIENTED_EDGE('',*,*,#2400,.F.);
#3283=ORIENTED_EDGE('',*,*,#2470,.T.);
#3284=ORIENTED_EDGE('',*,*,#2411,.F.);
#3285=ORIENTED_EDGE('',*,*,#2408,.T.);
#3286=ORIENTED_EDGE('',*,*,#2449,.T.);
#3287=ORIENTED_EDGE('',*,*,#2395,.T.);
#3288=ORIENTED_EDGE('',*,*,#2391,.F.);
#3289=ORIENTED_EDGE('',*,*,#2471,.T.);
#3290=ORIENTED_EDGE('',*,*,#2402,.F.);
#3291=ORIENTED_EDGE('',*,*,#2472,.T.);
#3292=ORIENTED_EDGE('',*,*,#2473,.T.);
#3293=ORIENTED_EDGE('',*,*,#2474,.T.);
#3294=ORIENTED_EDGE('',*,*,#2467,.T.);
#3295=ORIENTED_EDGE('',*,*,#2475,.T.);
#3296=ORIENTED_EDGE('',*,*,#2473,.F.);
#3297=ORIENTED_EDGE('',*,*,#2456,.F.);
#3298=ORIENTED_EDGE('',*,*,#2421,.F.);
#3299=ORIENTED_EDGE('',*,*,#2459,.F.);
#3300=ORIENTED_EDGE('',*,*,#2412,.F.);
#3301=ORIENTED_EDGE('',*,*,#2470,.F.);
#3302=ORIENTED_EDGE('',*,*,#2403,.F.);
#3303=ORIENTED_EDGE('',*,*,#2471,.F.);
#3304=ORIENTED_EDGE('',*,*,#2394,.F.);
#3305=ORIENTED_EDGE('',*,*,#2476,.T.);
#3306=ORIENTED_EDGE('',*,*,#2477,.T.);
#3307=ORIENTED_EDGE('',*,*,#2472,.F.);
#3308=ORIENTED_EDGE('',*,*,#2478,.F.);
#3309=ORIENTED_EDGE('',*,*,#2463,.F.);
#3310=ORIENTED_EDGE('',*,*,#2469,.F.);
#3311=ORIENTED_EDGE('',*,*,#2479,.F.);
#3312=ORIENTED_EDGE('',*,*,#2465,.F.);
#3313=ORIENTED_EDGE('',*,*,#2477,.F.);
#3314=ORIENTED_EDGE('',*,*,#2480,.T.);
#3315=ORIENTED_EDGE('',*,*,#2455,.F.);
#3316=ORIENTED_EDGE('',*,*,#2480,.F.);
#3317=ORIENTED_EDGE('',*,*,#2476,.F.);
#3318=ORIENTED_EDGE('',*,*,#2481,.T.);
#3319=ORIENTED_EDGE('',*,*,#2454,.F.);
#3320=ORIENTED_EDGE('',*,*,#2481,.F.);
#3321=ORIENTED_EDGE('',*,*,#2475,.F.);
#3322=ORIENTED_EDGE('',*,*,#2466,.T.);
#3323=ORIENTED_EDGE('',*,*,#2479,.T.);
#3324=ORIENTED_EDGE('',*,*,#2464,.T.);
#3325=ORIENTED_EDGE('',*,*,#2478,.T.);
#3326=ORIENTED_EDGE('',*,*,#2468,.T.);
#3327=ORIENTED_EDGE('',*,*,#2474,.F.);
#3328=ORIENTED_EDGE('',*,*,#2482,.T.);
#3329=ORIENTED_EDGE('',*,*,#2453,.F.);
#3330=ORIENTED_EDGE('',*,*,#2482,.F.);
#4159=CONICAL_SURFACE('',#4752,5.4,0.785398163397448);
#4160=CONICAL_SURFACE('',#4755,2.9,0.785398163397448);
#4161=CONICAL_SURFACE('',#4760,5.4,0.785398163397448);
#4162=CONICAL_SURFACE('',#4765,2.9,0.785398163397448);
#4163=CONICAL_SURFACE('',#4780,2.85,0.785398163397448);
#4164=CONICAL_SURFACE('',#4782,5.35,0.785398163397448);
#4165=CONICAL_SURFACE('',#4790,2.85,0.785398163397448);
#4166=CONICAL_SURFACE('',#4792,5.35,0.785398163397448);
#4167=CONICAL_SURFACE('',#4794,3.16,0.785398163397447);
#4263=ADVANCED_FACE('',(#596),#353,.T.);
#4264=ADVANCED_FACE('',(#597),#354,.T.);
#4265=ADVANCED_FACE('',(#598),#355,.T.);
#4266=ADVANCED_FACE('',(#599),#356,.T.);
#4267=ADVANCED_FACE('',(#600),#357,.T.);
#4268=ADVANCED_FACE('',(#601),#358,.T.);
#4269=ADVANCED_FACE('',(#602),#359,.T.);
#4270=ADVANCED_FACE('',(#603),#360,.T.);
#4271=ADVANCED_FACE('',(#604),#361,.T.);
#4272=ADVANCED_FACE('',(#605),#4159,.T.);
#4273=ADVANCED_FACE('',(#606),#4160,.T.);
#4274=ADVANCED_FACE('',(#607),#362,.T.);
#4275=ADVANCED_FACE('',(#608),#363,.T.);
#4276=ADVANCED_FACE('',(#609),#4161,.T.);
#4277=ADVANCED_FACE('',(#610),#364,.T.);
#4278=ADVANCED_FACE('',(#611),#4162,.T.);
#4279=ADVANCED_FACE('',(#612),#447,.T.);
#4280=ADVANCED_FACE('',(#613),#448,.T.);
#4281=ADVANCED_FACE('',(#614),#449,.T.);
#4282=ADVANCED_FACE('',(#615),#450,.T.);
#4283=ADVANCED_FACE('',(#616,#300,#301,#302),#365,.F.);
#4284=ADVANCED_FACE('',(#617),#4163,.T.);
#4285=ADVANCED_FACE('',(#618),#4164,.T.);
#4286=ADVANCED_FACE('',(#619),#451,.T.);
#4287=ADVANCED_FACE('',(#620),#452,.F.);
#4288=ADVANCED_FACE('',(#621),#4165,.T.);
#4289=ADVANCED_FACE('',(#622),#4166,.T.);
#4290=ADVANCED_FACE('',(#623),#4167,.F.);
#4291=ADVANCED_FACE('',(#624,#303,#304,#305),#366,.T.);
#4292=ADVANCED_FACE('',(#625),#367,.T.);
#4293=ADVANCED_FACE('',(#626),#368,.T.);
#4294=ADVANCED_FACE('',(#627),#453,.F.);
#4295=ADVANCED_FACE('',(#628),#454,.F.);
#4296=ADVANCED_FACE('',(#629),#455,.F.);
#4465=CLOSED_SHELL('',(#4263,#4264,#4265,#4266,#4267,#4268,#4269,#4270,
#4271,#4272,#4273,#4274,#4275,#4276,#4277,#4278,#4279,#4280,#4281,#4282,
#4283,#4284,#4285,#4286,#4287,#4288,#4289,#4290,#4291,#4292,#4293,#4294,
#4295,#4296));
#4742=AXIS2_PLACEMENT_3D('',#6610,#5425,#5426);
#4743=AXIS2_PLACEMENT_3D('',#6611,#5427,#5428);
#4744=AXIS2_PLACEMENT_3D('',#6624,#5431,#5432);
#4745=AXIS2_PLACEMENT_3D('',#6638,#5436,#5437);
#4746=AXIS2_PLACEMENT_3D('',#6651,#5440,#5441);
#4747=AXIS2_PLACEMENT_3D('',#6665,#5445,#5446);
#4748=AXIS2_PLACEMENT_3D('',#6678,#5449,#5450);
#4749=AXIS2_PLACEMENT_3D('',#6692,#5454,#5455);
#4750=AXIS2_PLACEMENT_3D('',#6705,#5458,#5459);
#4751=AXIS2_PLACEMENT_3D('',#6719,#5463,#5464);
#4752=AXIS2_PLACEMENT_3D('',#6731,#5466,#5467);
#4753=AXIS2_PLACEMENT_3D('',#6733,#5468,#5469);
#4754=AXIS2_PLACEMENT_3D('',#6738,#5470,#5471);
#4755=AXIS2_PLACEMENT_3D('',#6739,#5472,#5473);
#4756=AXIS2_PLACEMENT_3D('',#6740,#5474,#5475);
#4757=AXIS2_PLACEMENT_3D('',#6747,#5476,#5477);
#4758=AXIS2_PLACEMENT_3D('',#6752,#5478,#5479);
#4759=AXIS2_PLACEMENT_3D('',#6754,#5481,#5482);
#4760=AXIS2_PLACEMENT_3D('',#6761,#5484,#5485);
#4761=AXIS2_PLACEMENT_3D('',#6763,#5486,#5487);
#4762=AXIS2_PLACEMENT_3D('',#6764,#5488,#5489);
#4763=AXIS2_PLACEMENT_3D('',#6766,#5490,#5491);
#4764=AXIS2_PLACEMENT_3D('',#6771,#5492,#5493);
#4765=AXIS2_PLACEMENT_3D('',#6778,#5495,#5496);
#4766=AXIS2_PLACEMENT_3D('',#6779,#5497,#5498);
#4767=AXIS2_PLACEMENT_3D('',#6780,#5499,#5500);
#4768=AXIS2_PLACEMENT_3D('',#6781,#5501,#5502);
#4769=AXIS2_PLACEMENT_3D('',#6782,#5503,#5504);
#4770=AXIS2_PLACEMENT_3D('',#6783,#5505,#5506);
#4771=AXIS2_PLACEMENT_3D('',#6784,#5507,#5508);
#4772=AXIS2_PLACEMENT_3D('',#6785,#5509,#5510);
#4773=AXIS2_PLACEMENT_3D('',#6804,#5511,#5512);
#4774=AXIS2_PLACEMENT_3D('',#6805,#5513,#5514);
#4775=AXIS2_PLACEMENT_3D('',#6806,#5515,#5516);
#4776=AXIS2_PLACEMENT_3D('',#6807,#5517,#5518);
#4777=AXIS2_PLACEMENT_3D('',#6809,#5519,#5520);
#4778=AXIS2_PLACEMENT_3D('',#6811,#5521,#5522);
#4779=AXIS2_PLACEMENT_3D('',#6813,#5523,#5524);
#4780=AXIS2_PLACEMENT_3D('',#6814,#5525,#5526);
#4781=AXIS2_PLACEMENT_3D('',#6815,#5527,#5528);
#4782=AXIS2_PLACEMENT_3D('',#6816,#5529,#5530);
#4783=AXIS2_PLACEMENT_3D('',#6828,#5531,#5532);
#4784=AXIS2_PLACEMENT_3D('',#6829,#5533,#5534);
#4785=AXIS2_PLACEMENT_3D('',#6830,#5535,#5536);
#4786=AXIS2_PLACEMENT_3D('',#6850,#5537,#5538);
#4787=AXIS2_PLACEMENT_3D('',#6854,#5540,#5541);
#4788=AXIS2_PLACEMENT_3D('',#6871,#5542,#5543);
#4789=AXIS2_PLACEMENT_3D('',#6897,#5544,#5545);
#4790=AXIS2_PLACEMENT_3D('',#6898,#5546,#5547);
#4791=AXIS2_PLACEMENT_3D('',#6899,#5548,#5549);
#4792=AXIS2_PLACEMENT_3D('',#6900,#5550,#5551);
#4793=AXIS2_PLACEMENT_3D('',#6901,#5552,#5553);
#4794=AXIS2_PLACEMENT_3D('',#6902,#5554,#5555);
#4795=AXIS2_PLACEMENT_3D('',#6904,#5556,#5557);
#4796=AXIS2_PLACEMENT_3D('',#6907,#5559,#5560);
#4797=AXIS2_PLACEMENT_3D('',#6908,#5561,#5562);
#4798=AXIS2_PLACEMENT_3D('',#6909,#5563,#5564);
#4799=AXIS2_PLACEMENT_3D('',#6911,#5565,#5566);
#4800=AXIS2_PLACEMENT_3D('',#6913,#5567,#5568);
#4801=AXIS2_PLACEMENT_3D('',#6914,#5569,#5570);
#4802=AXIS2_PLACEMENT_3D('',#6916,#5572,#5573);
#4803=AXIS2_PLACEMENT_3D('',#6918,#5575,#5576);
#4804=AXIS2_PLACEMENT_3D('',#6920,#5578,#5579);
#4805=AXIS2_PLACEMENT_3D('',#6922,#5581,#5582);
#5425=DIRECTION('axis',(0.,0.,1.));
#5426=DIRECTION('refdir',(1.,0.,0.));
#5427=DIRECTION('center_axis',(0.,-0.707106781186548,0.707106781186548));
#5428=DIRECTION('ref_axis',(1.,0.,0.));
#5429=DIRECTION('',(1.,0.,0.));
#5430=DIRECTION('',(-1.,0.,0.));
#5431=DIRECTION('center_axis',(0.,-1.,0.));
#5432=DIRECTION('ref_axis',(1.,0.,0.));
#5433=DIRECTION('',(0.,0.,1.));
#5434=DIRECTION('',(-1.,0.,0.));
#5435=DIRECTION('',(0.,0.,1.));
#5436=DIRECTION('center_axis',(0.,-0.707106781186548,0.707106781186548));
#5437=DIRECTION('ref_axis',(1.,0.,0.));
#5438=DIRECTION('',(1.,0.,0.));
#5439=DIRECTION('',(-1.,0.,0.));
#5440=DIRECTION('center_axis',(0.,-1.,0.));
#5441=DIRECTION('ref_axis',(1.,0.,0.));
#5442=DIRECTION('',(0.,0.,1.));
#5443=DIRECTION('',(-1.,0.,0.));
#5444=DIRECTION('',(0.,0.,1.));
#5445=DIRECTION('center_axis',(0.,0.707106781186548,0.707106781186548));
#5446=DIRECTION('ref_axis',(1.,0.,0.));
#5447=DIRECTION('',(-1.,0.,0.));
#5448=DIRECTION('',(1.,0.,0.));
#5449=DIRECTION('center_axis',(0.,1.,0.));
#5450=DIRECTION('ref_axis',(-1.,0.,0.));
#5451=DIRECTION('',(0.,0.,1.));
#5452=DIRECTION('',(1.,0.,0.));
#5453=DIRECTION('',(0.,0.,1.));
#5454=DIRECTION('center_axis',(0.,0.707106781186548,0.707106781186548));
#5455=DIRECTION('ref_axis',(1.,0.,0.));
#5456=DIRECTION('',(-1.,0.,0.));
#5457=DIRECTION('',(1.,0.,0.));
#5458=DIRECTION('center_axis',(0.,1.,0.));
#5459=DIRECTION('ref_axis',(-1.,0.,0.));
#5460=DIRECTION('',(0.,0.,1.));
#5461=DIRECTION('',(1.,0.,0.));
#5462=DIRECTION('',(0.,0.,1.));
#5463=DIRECTION('center_axis',(0.,-0.707106781186548,-0.707106781186548));
#5464=DIRECTION('ref_axis',(-1.,0.,0.));
#5465=DIRECTION('',(1.,0.,0.));
#5466=DIRECTION('center_axis',(0.,0.,1.));
#5467=DIRECTION('ref_axis',(1.,0.,0.));
#5468=DIRECTION('center_axis',(0.,0.,1.));
#5469=DIRECTION('ref_axis',(1.,0.,0.));
#5470=DIRECTION('center_axis',(0.,0.,-1.));
#5471=DIRECTION('ref_axis',(1.,0.,0.));
#5472=DIRECTION('center_axis',(0.,0.,1.));
#5473=DIRECTION('ref_axis',(1.,0.,0.));
#5474=DIRECTION('center_axis',(0.,0.,-1.));
#5475=DIRECTION('ref_axis',(1.,0.,0.));
#5476=DIRECTION('center_axis',(0.,0.,1.));
#5477=DIRECTION('ref_axis',(1.,0.,0.));
#5478=DIRECTION('center_axis',(0.,-0.707106781186548,-0.707106781186548));
#5479=DIRECTION('ref_axis',(-1.,0.,0.));
#5480=DIRECTION('',(1.,0.,0.));
#5481=DIRECTION('center_axis',(0.,0.707106781186548,-0.707106781186548));
#5482=DIRECTION('ref_axis',(-1.,0.,0.));
#5483=DIRECTION('',(-1.,0.,0.));
#5484=DIRECTION('center_axis',(0.,0.,1.));
#5485=DIRECTION('ref_axis',(1.,0.,0.));
#5486=DIRECTION('center_axis',(0.,0.,-1.));
#5487=DIRECTION('ref_axis',(1.,0.,0.));
#5488=DIRECTION('center_axis',(0.,0.,-1.));
#5489=DIRECTION('ref_axis',(1.,0.,0.));
#5490=DIRECTION('center_axis',(0.,0.,1.));
#5491=DIRECTION('ref_axis',(1.,0.,0.));
#5492=DIRECTION('center_axis',(0.,0.707106781186548,-0.707106781186548));
#5493=DIRECTION('ref_axis',(-1.,0.,0.));
#5494=DIRECTION('',(-1.,0.,0.));
#5495=DIRECTION('center_axis',(0.,0.,1.));
#5496=DIRECTION('ref_axis',(-1.,0.,0.));
#5497=DIRECTION('center_axis',(0.,0.,-1.));
#5498=DIRECTION('ref_axis',(-1.,0.,0.));
#5499=DIRECTION('center_axis',(0.,0.,1.));
#5500=DIRECTION('ref_axis',(-1.,0.,0.));
#5501=DIRECTION('center_axis',(0.,0.,1.));
#5502=DIRECTION('ref_axis',(-1.,-3.21624529935327E-16,0.));
#5503=DIRECTION('center_axis',(0.,0.,1.));
#5504=DIRECTION('ref_axis',(-1.,0.,0.));
#5505=DIRECTION('center_axis',(0.,0.,1.));
#5506=DIRECTION('ref_axis',(1.,0.,0.));
#5507=DIRECTION('center_axis',(0.,0.,1.));
#5508=DIRECTION('ref_axis',(1.,0.,0.));
#5509=DIRECTION('center_axis',(0.,0.,1.));
#5510=DIRECTION('ref_axis',(1.,0.,0.));
#5511=DIRECTION('center_axis',(0.,0.,1.));
#5512=DIRECTION('ref_axis',(1.,0.,0.));
#5513=DIRECTION('center_axis',(0.,0.,1.));
#5514=DIRECTION('ref_axis',(1.,0.,0.));
#5515=DIRECTION('center_axis',(0.,0.,1.));
#5516=DIRECTION('ref_axis',(1.,0.,0.));
#5517=DIRECTION('center_axis',(0.,0.,1.));
#5518=DIRECTION('ref_axis',(1.,0.,0.));
#5519=DIRECTION('center_axis',(0.,0.,1.));
#5520=DIRECTION('ref_axis',(1.,0.,0.));
#5521=DIRECTION('center_axis',(0.,0.,1.));
#5522=DIRECTION('ref_axis',(1.,0.,0.));
#5523=DIRECTION('center_axis',(0.,0.,1.));
#5524=DIRECTION('ref_axis',(1.,0.,0.));
#5525=DIRECTION('center_axis',(0.,0.,-1.));
#5526=DIRECTION('ref_axis',(1.,0.,0.));
#5527=DIRECTION('center_axis',(0.,0.,-1.));
#5528=DIRECTION('ref_axis',(1.,0.,0.));
#5529=DIRECTION('center_axis',(0.,0.,-1.));
#5530=DIRECTION('ref_axis',(1.,0.,0.));
#5531=DIRECTION('center_axis',(0.,0.,1.));
#5532=DIRECTION('ref_axis',(1.,0.,0.));
#5533=DIRECTION('center_axis',(0.,0.,-1.));
#5534=DIRECTION('ref_axis',(1.,0.,0.));
#5535=DIRECTION('center_axis',(0.,0.,1.));
#5536=DIRECTION('ref_axis',(1.,0.,0.));
#5537=DIRECTION('center_axis',(0.,-1.,0.));
#5538=DIRECTION('ref_axis',(1.,0.,0.));
#5539=DIRECTION('',(0.,-1.,0.));
#5540=DIRECTION('center_axis',(0.,-1.,0.));
#5541=DIRECTION('ref_axis',(1.,0.,0.));
#5542=DIRECTION('center_axis',(0.,-1.,0.));
#5543=DIRECTION('ref_axis',(1.,0.,0.));
#5544=DIRECTION('center_axis',(0.,-1.,0.));
#5545=DIRECTION('ref_axis',(1.,0.,0.));
#5546=DIRECTION('center_axis',(0.,0.,-1.));
#5547=DIRECTION('ref_axis',(-1.,0.,0.));
#5548=DIRECTION('center_axis',(0.,0.,-1.));
#5549=DIRECTION('ref_axis',(-1.,0.,0.));
#5550=DIRECTION('center_axis',(0.,0.,-1.));
#5551=DIRECTION('ref_axis',(1.,0.,0.));
#5552=DIRECTION('center_axis',(0.,0.,-1.));
#5553=DIRECTION('ref_axis',(1.,0.,0.));
#5554=DIRECTION('center_axis',(0.,0.,1.));
#5555=DIRECTION('ref_axis',(1.,0.,0.));
#5556=DIRECTION('center_axis',(0.,0.,1.));
#5557=DIRECTION('ref_axis',(1.,0.,0.));
#5558=DIRECTION('',(0.707106781186547,8.65956056235492E-17,-0.707106781186548));
#5559=DIRECTION('center_axis',(0.,0.,-1.));
#5560=DIRECTION('ref_axis',(1.,0.,0.));
#5561=DIRECTION('center_axis',(0.,0.,-1.));
#5562=DIRECTION('ref_axis',(1.,0.,0.));
#5563=DIRECTION('center_axis',(0.,0.,1.));
#5564=DIRECTION('ref_axis',(1.,0.,0.));
#5565=DIRECTION('center_axis',(0.,0.,-1.));
#5566=DIRECTION('ref_axis',(1.,0.,0.));
#5567=DIRECTION('center_axis',(0.,0.,-1.));
#5568=DIRECTION('ref_axis',(1.,0.,0.));
#5569=DIRECTION('center_axis',(0.,1.,0.));
#5570=DIRECTION('ref_axis',(1.,0.,0.));
#5571=DIRECTION('',(0.,0.,1.));
#5572=DIRECTION('center_axis',(0.,1.,0.));
#5573=DIRECTION('ref_axis',(1.,0.,0.));
#5574=DIRECTION('',(0.,0.,-1.));
#5575=DIRECTION('center_axis',(0.,0.,-1.));
#5576=DIRECTION('ref_axis',(1.,0.,0.));
#5577=DIRECTION('',(0.,0.,-1.));
#5578=DIRECTION('center_axis',(0.,0.,-1.));
#5579=DIRECTION('ref_axis',(1.,0.,0.));
#5580=DIRECTION('',(0.,0.,-1.));
#5581=DIRECTION('center_axis',(0.,0.,-1.));
#5582=DIRECTION('ref_axis',(1.,0.,0.));
#5583=DIRECTION('',(0.,0.,-1.));
#6610=CARTESIAN_POINT('',(0.,0.,0.));
#6611=CARTESIAN_POINT('Origin',(2.47436860633172,-2.3,11.9));
#6612=CARTESIAN_POINT('',(4.7116875957559,-2.2,12.));
#6613=CARTESIAN_POINT('',(4.83735464897913,-2.4,11.8));
#6614=CARTESIAN_POINT('Ctrl Pts',(4.83735464897913,-2.4,11.8));
#6615=CARTESIAN_POINT('Ctrl Pts',(4.77452112236735,-2.29868398264425,11.9013160173557));
#6616=CARTESIAN_POINT('Ctrl Pts',(4.7116875957559,-2.2,12.));
#6617=CARTESIAN_POINT('',(10.37211794039,-2.4,11.8));
#6618=CARTESIAN_POINT('',(2.47436860633172,-2.4,11.8));
#6619=CARTESIAN_POINT('',(10.4347524157501,-2.2,12.));
#6620=CARTESIAN_POINT('Ctrl Pts',(10.4347524157501,-2.2,12.));
#6621=CARTESIAN_POINT('Ctrl Pts',(10.4034351780701,-2.29803846124815,11.9019615387518));
#6622=CARTESIAN_POINT('Ctrl Pts',(10.37211794039,-2.4,11.8));
#6623=CARTESIAN_POINT('',(2.47436860633172,-2.2,12.));
#6624=CARTESIAN_POINT('Origin',(4.94873721266345,-2.4,9.5));
#6625=CARTESIAN_POINT('',(4.94873721266345,-2.4,11.7));
#6626=CARTESIAN_POINT('Ctrl Pts',(4.83735464897798,-2.4,11.800000000001));
#6627=CARTESIAN_POINT('Ctrl Pts',(4.89253500162966,-2.4,11.7505690860322));
#6628=CARTESIAN_POINT('Ctrl Pts',(4.94873721266345,-2.4,11.7));
#6629=CARTESIAN_POINT('',(4.94873721266345,-2.4,9.7));
#6630=CARTESIAN_POINT('',(4.94873721266345,-2.4,9.5));
#6631=CARTESIAN_POINT('',(10.2,-2.4,9.7));
#6632=CARTESIAN_POINT('',(2.47436860633172,-2.4,9.7));
#6633=CARTESIAN_POINT('',(10.2,-2.4,11.7));
#6634=CARTESIAN_POINT('',(10.2,-2.4,9.5));
#6635=CARTESIAN_POINT('Ctrl Pts',(10.2,-2.4,11.7));
#6636=CARTESIAN_POINT('Ctrl Pts',(10.2875175968085,-2.4,11.7525105580851));
#6637=CARTESIAN_POINT('Ctrl Pts',(10.37211794039,-2.4,11.8));
#6638=CARTESIAN_POINT('Origin',(-5.1,-2.3,11.9));
#6639=CARTESIAN_POINT('',(-10.4347524157501,-2.2,12.));
#6640=CARTESIAN_POINT('',(-10.37211794039,-2.4,11.8));
#6641=CARTESIAN_POINT('Ctrl Pts',(-10.37211794039,-2.4,11.8));
#6642=CARTESIAN_POINT('Ctrl Pts',(-10.4034351780701,-2.29803846124801,11.901961538752));
#6643=CARTESIAN_POINT('Ctrl Pts',(-10.4347524157501,-2.2,12.));
#6644=CARTESIAN_POINT('',(-4.83735464897913,-2.4,11.8));
#6645=CARTESIAN_POINT('',(-5.1,-2.4,11.8));
#6646=CARTESIAN_POINT('',(-4.7116875957559,-2.2,12.));
#6647=CARTESIAN_POINT('Ctrl Pts',(-4.7116875957559,-2.2,12.));
#6648=CARTESIAN_POINT('Ctrl Pts',(-4.7745211223673,-2.29868398264418,11.9013160173558));
#6649=CARTESIAN_POINT('Ctrl Pts',(-4.83735464897913,-2.4,11.8));
#6650=CARTESIAN_POINT('',(-5.1,-2.2,12.));
#6651=CARTESIAN_POINT('Origin',(-10.2,-2.4,9.5));
#6652=CARTESIAN_POINT('',(-10.2,-2.4,11.7));
#6653=CARTESIAN_POINT('Ctrl Pts',(-10.37211794039,-2.4,11.8));
#6654=CARTESIAN_POINT('Ctrl Pts',(-10.2875175968085,-2.4,11.7525105580851));
#6655=CARTESIAN_POINT('Ctrl Pts',(-10.2,-2.4,11.7));
#6656=CARTESIAN_POINT('',(-10.2,-2.4,9.7));
#6657=CARTESIAN_POINT('',(-10.2,-2.4,9.5));
#6658=CARTESIAN_POINT('',(-4.94873721266345,-2.4,9.7));
#6659=CARTESIAN_POINT('',(-5.1,-2.4,9.7));
#6660=CARTESIAN_POINT('',(-4.94873721266345,-2.4,11.7));
#6661=CARTESIAN_POINT('',(-4.94873721266345,-2.4,9.5));
#6662=CARTESIAN_POINT('Ctrl Pts',(-4.94873721266345,-2.4,11.7));
#6663=CARTESIAN_POINT('Ctrl Pts',(-4.89253500163078,-2.4,11.7505690860312));
#6664=CARTESIAN_POINT('Ctrl Pts',(-4.83735464898018,-2.4,11.7999999999991));
#6665=CARTESIAN_POINT('Origin',(-2.47436860633172,2.3,11.9));
#6666=CARTESIAN_POINT('',(-4.7116875957559,2.2,12.));
#6667=CARTESIAN_POINT('',(-4.83735464897913,2.4,11.8));
#6668=CARTESIAN_POINT('Ctrl Pts',(-4.83735464897913,2.4,11.8));
#6669=CARTESIAN_POINT('Ctrl Pts',(-4.7745211223673,2.29868398264418,11.9013160173558));
#6670=CARTESIAN_POINT('Ctrl Pts',(-4.7116875957559,2.2,12.));
#6671=CARTESIAN_POINT('',(-10.37211794039,2.4,11.8));
#6672=CARTESIAN_POINT('',(-2.47436860633172,2.4,11.8));
#6673=CARTESIAN_POINT('',(-10.4347524157501,2.2,12.));
#6674=CARTESIAN_POINT('Ctrl Pts',(-10.4347524157501,2.2,12.));
#6675=CARTESIAN_POINT('Ctrl Pts',(-10.4034351780701,2.29803846124801,11.901961538752));
#6676=CARTESIAN_POINT('Ctrl Pts',(-10.37211794039,2.4,11.8));
#6677=CARTESIAN_POINT('',(-2.47436860633172,2.2,12.));
#6678=CARTESIAN_POINT('Origin',(-4.94873721266345,2.4,9.5));
#6679=CARTESIAN_POINT('',(-4.94873721266345,2.4,11.7));
#6680=CARTESIAN_POINT('Ctrl Pts',(-4.83735464897788,2.4,11.8000000000011));
#6681=CARTESIAN_POINT('Ctrl Pts',(-4.89253500162949,2.4,11.7505690860323));
#6682=CARTESIAN_POINT('Ctrl Pts',(-4.94873721266345,2.4,11.7));
#6683=CARTESIAN_POINT('',(-4.94873721266345,2.4,9.7));
#6684=CARTESIAN_POINT('',(-4.94873721266345,2.4,9.5));
#6685=CARTESIAN_POINT('',(-10.2,2.4,9.7));
#6686=CARTESIAN_POINT('',(-2.47436860633172,2.4,9.7));
#6687=CARTESIAN_POINT('',(-10.2,2.4,11.7));
#6688=CARTESIAN_POINT('',(-10.2,2.4,9.5));
#6689=CARTESIAN_POINT('Ctrl Pts',(-10.2,2.4,11.7));
#6690=CARTESIAN_POINT('Ctrl Pts',(-10.2875175968085,2.4,11.7525105580851));
#6691=CARTESIAN_POINT('Ctrl Pts',(-10.37211794039,2.4,11.8));
#6692=CARTESIAN_POINT('Origin',(5.1,2.3,11.9));
#6693=CARTESIAN_POINT('',(10.4347524157501,2.2,12.));
#6694=CARTESIAN_POINT('',(10.37211794039,2.4,11.8));
#6695=CARTESIAN_POINT('Ctrl Pts',(10.37211794039,2.4,11.8));
#6696=CARTESIAN_POINT('Ctrl Pts',(10.4034351780701,2.29803846124801,11.901961538752));
#6697=CARTESIAN_POINT('Ctrl Pts',(10.4347524157501,2.2,12.));
#6698=CARTESIAN_POINT('',(4.83735464897913,2.4,11.8));
#6699=CARTESIAN_POINT('',(5.1,2.4,11.8));
#6700=CARTESIAN_POINT('',(4.7116875957559,2.2,12.));
#6701=CARTESIAN_POINT('Ctrl Pts',(4.7116875957559,2.2,12.));
#6702=CARTESIAN_POINT('Ctrl Pts',(4.7745211223673,2.29868398264418,11.9013160173558));
#6703=CARTESIAN_POINT('Ctrl Pts',(4.83735464897913,2.4,11.8));
#6704=CARTESIAN_POINT('',(5.1,2.2,12.));
#6705=CARTESIAN_POINT('Origin',(10.2,2.4,9.5));
#6706=CARTESIAN_POINT('',(10.2,2.4,11.7));
#6707=CARTESIAN_POINT('Ctrl Pts',(10.37211794039,2.4,11.8));
#6708=CARTESIAN_POINT('Ctrl Pts',(10.2875175968085,2.4,11.7525105580851));
#6709=CARTESIAN_POINT('Ctrl Pts',(10.2,2.4,11.7));
#6710=CARTESIAN_POINT('',(10.2,2.4,9.7));
#6711=CARTESIAN_POINT('',(10.2,2.4,9.5));
#6712=CARTESIAN_POINT('',(4.94873721266345,2.4,9.7));
#6713=CARTESIAN_POINT('',(5.1,2.4,9.7));
#6714=CARTESIAN_POINT('',(4.94873721266345,2.4,11.7));
#6715=CARTESIAN_POINT('',(4.94873721266345,2.4,9.5));
#6716=CARTESIAN_POINT('Ctrl Pts',(4.94873721497344,2.4,11.6999999979215));
#6717=CARTESIAN_POINT('Ctrl Pts',(4.89253500276439,2.4,11.7505690850157));
#6718=CARTESIAN_POINT('Ctrl Pts',(4.83735464898018,2.4,11.7999999999991));
#6719=CARTESIAN_POINT('Origin',(-5.1,-2.3,9.6));
#6720=CARTESIAN_POINT('',(-10.2679491924311,-2.2,9.5));
#6721=CARTESIAN_POINT('',(-4.82182538049648,-2.2,9.5));
#6722=CARTESIAN_POINT('',(-5.1,-2.2,9.5));
#6723=CARTESIAN_POINT('Ctrl Pts',(-4.82182538049648,-2.2,9.5));
#6724=CARTESIAN_POINT('Ctrl Pts',(-4.86458548124608,-2.26651023840872,9.56651023840872));
#6725=CARTESIAN_POINT('Ctrl Pts',(-4.90689191151574,-2.33319954872105,9.63319954872104));
#6726=CARTESIAN_POINT('Ctrl Pts',(-4.94873721266345,-2.4,9.7));
#6727=CARTESIAN_POINT('Ctrl Pts',(-10.2679491924311,-2.2,9.5));
#6728=CARTESIAN_POINT('Ctrl Pts',(-10.2448893867531,-2.26656792507827,9.56656792507827));
#6729=CARTESIAN_POINT('Ctrl Pts',(-10.2222358749559,-2.3332923751323,9.6332923751323));
#6730=CARTESIAN_POINT('Ctrl Pts',(-10.2,-2.4,9.7));
#6731=CARTESIAN_POINT('Origin',(0.,0.,9.6));
#6732=CARTESIAN_POINT('',(4.82182538049648,-2.2,9.5));
#6733=CARTESIAN_POINT('Origin',(0.,0.,9.5));
#6734=CARTESIAN_POINT('Ctrl Pts',(4.82182538049648,-2.2,9.5));
#6735=CARTESIAN_POINT('Ctrl Pts',(4.86458548124613,-2.26651023840879,9.56651023840879));
#6736=CARTESIAN_POINT('Ctrl Pts',(4.90689191151583,-2.33319954872119,9.63319954872119));
#6737=CARTESIAN_POINT('Ctrl Pts',(4.94873721266345,-2.4,9.7));
#6738=CARTESIAN_POINT('Origin',(0.,0.,9.7));
#6739=CARTESIAN_POINT('Origin',(12.,0.,9.6));
#6740=CARTESIAN_POINT('Origin',(12.,0.,9.7));
#6741=CARTESIAN_POINT('',(10.2679491924311,-2.2,9.5));
#6742=CARTESIAN_POINT('Ctrl Pts',(10.2,-2.4,9.7));
#6743=CARTESIAN_POINT('Ctrl Pts',(10.2222358749557,-2.33329237513297,9.63329237513297));
#6744=CARTESIAN_POINT('Ctrl Pts',(10.244889386753,-2.26656792507858,9.56656792507857));
#6745=CARTESIAN_POINT('Ctrl Pts',(10.2679491924311,-2.2,9.5));
#6746=CARTESIAN_POINT('',(10.2679491924311,2.2,9.5));
#6747=CARTESIAN_POINT('Origin',(12.,0.,9.5));
#6748=CARTESIAN_POINT('Ctrl Pts',(10.2679491924311,2.2,9.5));
#6749=CARTESIAN_POINT('Ctrl Pts',(10.2448893867531,2.26656792507827,9.56656792507827));
#6750=CARTESIAN_POINT('Ctrl Pts',(10.2222358749559,2.3332923751323,9.6332923751323));
#6751=CARTESIAN_POINT('Ctrl Pts',(10.2,2.4,9.7));
#6752=CARTESIAN_POINT('Origin',(2.47436860633172,-2.3,9.6));
#6753=CARTESIAN_POINT('',(2.47436860633172,-2.2,9.5));
#6754=CARTESIAN_POINT('Origin',(5.1,2.3,9.6));
#6755=CARTESIAN_POINT('',(4.82182538049648,2.2,9.5));
#6756=CARTESIAN_POINT('',(5.1,2.2,9.5));
#6757=CARTESIAN_POINT('Ctrl Pts',(4.82182538049648,2.2,9.5));
#6758=CARTESIAN_POINT('Ctrl Pts',(4.86458548124611,2.26651023840876,9.56651023840876));
#6759=CARTESIAN_POINT('Ctrl Pts',(4.90689191151579,2.33319954872112,9.63319954872112));
#6760=CARTESIAN_POINT('Ctrl Pts',(4.94873721266345,2.4,9.7));
#6761=CARTESIAN_POINT('Origin',(0.,0.,9.6));
#6762=CARTESIAN_POINT('',(0.,5.5,9.7));
#6763=CARTESIAN_POINT('Origin',(0.,0.,9.7));
#6764=CARTESIAN_POINT('Origin',(0.,0.,9.7));
#6765=CARTESIAN_POINT('',(-4.82182538049648,2.2,9.5));
#6766=CARTESIAN_POINT('Origin',(0.,0.,9.5));
#6767=CARTESIAN_POINT('Ctrl Pts',(-4.82182538049648,2.2,9.5));
#6768=CARTESIAN_POINT('Ctrl Pts',(-4.86458548124609,2.26651023840874,9.56651023840873));
#6769=CARTESIAN_POINT('Ctrl Pts',(-4.90689191151576,2.33319954872108,9.63319954872108));
#6770=CARTESIAN_POINT('Ctrl Pts',(-4.94873721266345,2.4,9.7));
#6771=CARTESIAN_POINT('Origin',(-2.47436860633172,2.3,9.6));
#6772=CARTESIAN_POINT('',(-10.2679491924311,2.2,9.5));
#6773=CARTESIAN_POINT('',(-2.47436860633172,2.2,9.5));
#6774=CARTESIAN_POINT('Ctrl Pts',(-10.2679491924311,2.2,9.5));
#6775=CARTESIAN_POINT('Ctrl Pts',(-10.244889386753,2.26656792507857,9.56656792507857));
#6776=CARTESIAN_POINT('Ctrl Pts',(-10.2222358749557,2.33329237513297,9.63329237513297));
#6777=CARTESIAN_POINT('Ctrl Pts',(-10.2,2.4,9.7));
#6778=CARTESIAN_POINT('Origin',(-12.,0.,9.6));
#6779=CARTESIAN_POINT('Origin',(-12.,0.,9.7));
#6780=CARTESIAN_POINT('Origin',(-12.,0.,9.5));
#6781=CARTESIAN_POINT('Origin',(-12.,0.,9.5));
#6782=CARTESIAN_POINT('Origin',(-12.,0.,11.7));
#6783=CARTESIAN_POINT('Origin',(0.,0.,9.5));
#6784=CARTESIAN_POINT('Origin',(0.,0.,11.7));
#6785=CARTESIAN_POINT('Origin',(0.,0.,9.5));
#6786=CARTESIAN_POINT('',(0.447213604330343,5.4817880287459,11.6999999979215));
#6787=CARTESIAN_POINT('Ctrl Pts',(-1.04083408558608E-16,5.5,9.7));
#6788=CARTESIAN_POINT('Ctrl Pts',(0.132186811917676,5.5,9.7));
#6789=CARTESIAN_POINT('Ctrl Pts',(0.272965016647602,5.49475196102956,9.72648386715131));
#6790=CARTESIAN_POINT('Ctrl Pts',(0.531569703786443,5.47578694476791,9.83374194918294));
#6791=CARTESIAN_POINT('Ctrl Pts',(0.649422667404825,5.4623316644562,9.91449842691308));
#6792=CARTESIAN_POINT('Ctrl Pts',(0.835505886786072,5.43697965273112,10.1005816462943));
#6793=CARTESIAN_POINT('Ctrl Pts',(0.91625898403177,5.42341568535631,10.2184327722933));
#6794=CARTESIAN_POINT('Ctrl Pts',(1.02351461335488,5.40420078323371,10.4770310937253));
#6795=CARTESIAN_POINT('Ctrl Pts',(1.05,5.39884246852971,10.6178070593475));
#6796=CARTESIAN_POINT('Ctrl Pts',(1.05,5.39884246852971,10.75));
#6797=CARTESIAN_POINT('Ctrl Pts',(1.05,5.39884246852971,10.8821929406525));
#6798=CARTESIAN_POINT('Ctrl Pts',(1.02351461335488,5.40420078323371,11.0229689062747));
#6799=CARTESIAN_POINT('Ctrl Pts',(0.91625898403177,5.42341568535631,11.2815672277067));
#6800=CARTESIAN_POINT('Ctrl Pts',(0.835505886786072,5.43697965273112,11.3994183537057));
#6801=CARTESIAN_POINT('Ctrl Pts',(0.660316211845406,5.46084752597609,11.5746080286463));
#6802=CARTESIAN_POINT('Ctrl Pts',(0.558936689613752,5.47267346917065,11.6474062234574));
#6803=CARTESIAN_POINT('Ctrl Pts',(0.447213603533743,5.48178802881089,11.6999999962181));
#6804=CARTESIAN_POINT('Origin',(0.,0.,11.7));
#6805=CARTESIAN_POINT('Origin',(12.,0.,9.5));
#6806=CARTESIAN_POINT('Origin',(12.,0.,11.7));
#6807=CARTESIAN_POINT('Origin',(0.,0.,9.5));
#6808=CARTESIAN_POINT('',(-3.01,-3.68618686543353E-16,9.5));
#6809=CARTESIAN_POINT('Origin',(0.,0.,9.5));
#6810=CARTESIAN_POINT('',(10.48,-1.86146313470398E-16,9.5));
#6811=CARTESIAN_POINT('Origin',(12.,0.,9.5));
#6812=CARTESIAN_POINT('',(-13.52,-1.86146313470398E-16,9.5));
#6813=CARTESIAN_POINT('Origin',(-12.,0.,9.5));
#6814=CARTESIAN_POINT('Origin',(12.,0.,11.85));
#6815=CARTESIAN_POINT('Origin',(12.,0.,12.));
#6816=CARTESIAN_POINT('Origin',(0.,0.,11.85));
#6817=CARTESIAN_POINT('',(-0.447213604330343,5.4817880287459,11.6999999979215));
#6818=CARTESIAN_POINT('Ctrl Pts',(0.447213602432565,5.4817880321751,11.6999999967365));
#6819=CARTESIAN_POINT('Ctrl Pts',(0.414910948534785,5.46916630571322,11.7152065085969));
#6820=CARTESIAN_POINT('Ctrl Pts',(0.381292409563767,5.45779439913161,11.7290076072377));
#6821=CARTESIAN_POINT('Ctrl Pts',(0.235875663864367,5.41607161270286,11.7798828268936));
#6822=CARTESIAN_POINT('Ctrl Pts',(0.114682100258675,5.4,11.8));
#6823=CARTESIAN_POINT('Ctrl Pts',(-0.114682100258675,5.4,11.8));
#6824=CARTESIAN_POINT('Ctrl Pts',(-0.235875663864366,5.41607161270286,11.7798828268936));
#6825=CARTESIAN_POINT('Ctrl Pts',(-0.381292409563766,5.45779439913161,11.7290076072377));
#6826=CARTESIAN_POINT('Ctrl Pts',(-0.414910948534784,5.46916630571322,11.7152065085969));
#6827=CARTESIAN_POINT('Ctrl Pts',(-0.447213602432565,5.4817880321751,11.6999999967365));
#6828=CARTESIAN_POINT('Origin',(0.,0.,11.7));
#6829=CARTESIAN_POINT('Origin',(0.,0.,12.));
#6830=CARTESIAN_POINT('Origin',(0.,0.,9.5));
#6831=CARTESIAN_POINT('',(-1.05,5.39884246852971,10.75));
#6832=CARTESIAN_POINT('Ctrl Pts',(-0.447213603533744,5.48178802881089,11.6999999962181));
#6833=CARTESIAN_POINT('Ctrl Pts',(-0.558936689613753,5.47267346917065,11.6474062234574));
#6834=CARTESIAN_POINT('Ctrl Pts',(-0.660316211845406,5.46084752597609,11.5746080286463));
#6835=CARTESIAN_POINT('Ctrl Pts',(-0.835505886786072,5.43697965273112,11.3994183537057));
#6836=CARTESIAN_POINT('Ctrl Pts',(-0.91625898403177,5.42341568535631,11.2815672277067));
#6837=CARTESIAN_POINT('Ctrl Pts',(-1.02351461335488,5.40420078323371,11.0229689062747));
#6838=CARTESIAN_POINT('Ctrl Pts',(-1.05,5.39884246852971,10.8821929406525));
#6839=CARTESIAN_POINT('Ctrl Pts',(-1.05,5.39884246852971,10.75));
#6840=CARTESIAN_POINT('Ctrl Pts',(-1.05,5.39884246852971,10.75));
#6841=CARTESIAN_POINT('Ctrl Pts',(-1.05,5.39884246852971,10.6178070593475));
#6842=CARTESIAN_POINT('Ctrl Pts',(-1.02351461335488,5.40420078323371,10.4770310937253));
#6843=CARTESIAN_POINT('Ctrl Pts',(-0.91625898403177,5.42341568535631,10.2184327722933));
#6844=CARTESIAN_POINT('Ctrl Pts',(-0.835505886786073,5.43697965273112,10.1005816462943));
#6845=CARTESIAN_POINT('Ctrl Pts',(-0.649422667404826,5.4623316644562,9.91449842691308));
#6846=CARTESIAN_POINT('Ctrl Pts',(-0.531569703786443,5.47578694476791,9.83374194918294));
#6847=CARTESIAN_POINT('Ctrl Pts',(-0.272965016647603,5.49475196102956,9.72648386715131));
#6848=CARTESIAN_POINT('Ctrl Pts',(-0.132186811917677,5.5,9.7));
#6849=CARTESIAN_POINT('Ctrl Pts',(-1.73472347597681E-16,5.5,9.7));
#6850=CARTESIAN_POINT('Origin',(0.,5.5,10.75));
#6851=CARTESIAN_POINT('',(-1.05,2.9,10.75));
#6852=CARTESIAN_POINT('',(-1.05,5.5,10.75));
#6853=CARTESIAN_POINT('',(-0.806287789812048,2.9,10.077393131168));
#6854=CARTESIAN_POINT('Origin',(0.,2.9,10.75));
#6855=CARTESIAN_POINT('',(0.806287789812048,2.9,10.077393131168));
#6856=CARTESIAN_POINT('Ctrl Pts',(0.806287789812047,2.9,10.077393131168));
#6857=CARTESIAN_POINT('Ctrl Pts',(0.785808654937835,2.90569381944655,10.0528437589267));
#6858=CARTESIAN_POINT('Ctrl Pts',(0.76444442856579,2.91139815952389,10.029520188074));
#6859=CARTESIAN_POINT('Ctrl Pts',(0.649888518401964,2.94055606794566,9.91496427791022));
#6860=CARTESIAN_POINT('Ctrl Pts',(0.53255794166538,2.96538003783021,9.83432362785116));
#6861=CARTESIAN_POINT('Ctrl Pts',(0.274166742773895,3.00032153730045,9.72681194070543));
#6862=CARTESIAN_POINT('Ctrl Pts',(0.133022354666825,3.01,9.7));
#6863=CARTESIAN_POINT('Ctrl Pts',(-0.133022354666825,3.01,9.7));
#6864=CARTESIAN_POINT('Ctrl Pts',(-0.274166742773895,3.00032153730045,9.72681194070543));
#6865=CARTESIAN_POINT('Ctrl Pts',(-0.53255794166538,2.96538003783021,9.83432362785116));
#6866=CARTESIAN_POINT('Ctrl Pts',(-0.649888518401964,2.94055606794566,9.91496427791022));
#6867=CARTESIAN_POINT('Ctrl Pts',(-0.76444442856579,2.91139815952389,10.029520188074));
#6868=CARTESIAN_POINT('Ctrl Pts',(-0.785808654937835,2.90569381944655,10.0528437589267));
#6869=CARTESIAN_POINT('Ctrl Pts',(-0.806287789812047,2.9,10.077393131168));
#6870=CARTESIAN_POINT('',(0.806287789812048,2.9,11.422606868832));
#6871=CARTESIAN_POINT('Origin',(0.,2.9,10.75));
#6872=CARTESIAN_POINT('',(0.44721360294724,2.97659200988966,11.6999999982471));
#6873=CARTESIAN_POINT('Ctrl Pts',(0.447213602284006,2.9765920099893,11.6999999968064));
#6874=CARTESIAN_POINT('Ctrl Pts',(0.559174059233342,2.9597706790519,11.6472944816127));
#6875=CARTESIAN_POINT('Ctrl Pts',(0.660473235012751,2.93786194070974,11.574451005479));
#6876=CARTESIAN_POINT('Ctrl Pts',(0.76444442856579,2.91139815952389,11.470479811926));
#6877=CARTESIAN_POINT('Ctrl Pts',(0.785808654937837,2.90569381944655,11.4471562410733));
#6878=CARTESIAN_POINT('Ctrl Pts',(0.806287789812047,2.9,11.422606868832));
#6879=CARTESIAN_POINT('',(-0.44721360294724,2.97659200988966,11.6999999982471));
#6880=CARTESIAN_POINT('Ctrl Pts',(-0.447213601060151,2.97659200752633,11.6999999973825));
#6881=CARTESIAN_POINT('Ctrl Pts',(-0.390045315290127,3.01239525686365,11.7269120342416));
#6882=CARTESIAN_POINT('Ctrl Pts',(-0.324286474226429,3.04489074102158,11.7512712452848));
#6883=CARTESIAN_POINT('Ctrl Pts',(-0.171947398222887,3.09567084784442,11.7892957080173));
#6884=CARTESIAN_POINT('Ctrl Pts',(-0.0834561363660907,3.11,11.8));
#6885=CARTESIAN_POINT('Ctrl Pts',(0.0834561363660904,3.11,11.8));
#6886=CARTESIAN_POINT('Ctrl Pts',(0.171947398222886,3.09567084784442,11.7892957080173));
#6887=CARTESIAN_POINT('Ctrl Pts',(0.324286474226428,3.04489074102158,11.7512712452848));
#6888=CARTESIAN_POINT('Ctrl Pts',(0.390045315290127,3.01239525686365,11.7269120342416));
#6889=CARTESIAN_POINT('Ctrl Pts',(0.447213601060151,2.97659200752634,11.6999999973825));
#6890=CARTESIAN_POINT('',(-0.806287789812048,2.9,11.422606868832));
#6891=CARTESIAN_POINT('Ctrl Pts',(-0.806287789812047,2.9,11.422606868832));
#6892=CARTESIAN_POINT('Ctrl Pts',(-0.785808654937835,2.90569381944655,11.4471562410733));
#6893=CARTESIAN_POINT('Ctrl Pts',(-0.76444442856579,2.91139815952389,11.470479811926));
#6894=CARTESIAN_POINT('Ctrl Pts',(-0.66047323501275,2.93786194070974,11.574451005479));
#6895=CARTESIAN_POINT('Ctrl Pts',(-0.559174059233342,2.9597706790519,11.6472944816127));
#6896=CARTESIAN_POINT('Ctrl Pts',(-0.447213602284006,2.9765920099893,11.6999999968064));
#6897=CARTESIAN_POINT('Origin',(0.,2.9,10.75));
#6898=CARTESIAN_POINT('Origin',(-12.,0.,11.85));
#6899=CARTESIAN_POINT('Origin',(-12.,0.,12.));
#6900=CARTESIAN_POINT('Origin',(0.,0.,11.85));
#6901=CARTESIAN_POINT('Origin',(0.,0.,12.));
#6902=CARTESIAN_POINT('Origin',(0.,0.,11.85));
#6903=CARTESIAN_POINT('',(-3.31,-4.05358090517774E-16,12.));
#6904=CARTESIAN_POINT('Origin',(0.,0.,12.));
#6905=CARTESIAN_POINT('',(-3.00999999738253,-3.68618686222806E-16,11.6999999973825));
#6906=CARTESIAN_POINT('',(-3.16,-3.86988388530564E-16,11.85));
#6907=CARTESIAN_POINT('Origin',(0.,0.,11.7));
#6908=CARTESIAN_POINT('Origin',(0.,0.,11.7));
#6909=CARTESIAN_POINT('Origin',(0.,0.,12.));
#6910=CARTESIAN_POINT('',(10.48,-1.86146313470398E-16,12.));
#6911=CARTESIAN_POINT('Origin',(12.,0.,12.));
#6912=CARTESIAN_POINT('',(-13.52,-1.86146313470398E-16,12.));
#6913=CARTESIAN_POINT('Origin',(-12.,0.,12.));
#6914=CARTESIAN_POINT('Origin',(0.,2.9,10.75));
#6915=CARTESIAN_POINT('',(-0.806287789812048,2.9,12.));
#6916=CARTESIAN_POINT('Origin',(0.,2.9,10.75));
#6917=CARTESIAN_POINT('',(0.806287789812048,2.9,12.));
#6918=CARTESIAN_POINT('Origin',(-12.,0.,12.));
#6919=CARTESIAN_POINT('',(-13.52,1.86146313470398E-16,12.));
#6920=CARTESIAN_POINT('Origin',(12.,0.,12.));
#6921=CARTESIAN_POINT('',(10.48,1.86146313470398E-16,12.));
#6922=CARTESIAN_POINT('Origin',(0.,0.,12.));
#6923=CARTESIAN_POINT('',(-3.01,3.68618686543353E-16,12.));
#11408=UNCERTAINTY_MEASURE_WITH_UNIT(LENGTH_MEASURE(0.01),#11431,
'DISTANCE_ACCURACY_VALUE',
'Maximum model space distance between geometric entities at asserted c
onnectivities');
#11416=UNCERTAINTY_MEASURE_WITH_UNIT(LENGTH_MEASURE(0.01),#11431,
'DISTANCE_ACCURACY_VALUE',
'Maximum model space distance between geometric entities at asserted c
onnectivities');
#11422=(
GEOMETRIC_REPRESENTATION_CONTEXT(3)
GLOBAL_UNCERTAINTY_ASSIGNED_CONTEXT((#11408))
GLOBAL_UNIT_ASSIGNED_CONTEXT((#11431,#11433,#11434))
REPRESENTATION_CONTEXT('','3D')
);
#11430=(
GEOMETRIC_REPRESENTATION_CONTEXT(3)
GLOBAL_UNCERTAINTY_ASSIGNED_CONTEXT((#11416))
GLOBAL_UNIT_ASSIGNED_CONTEXT((#11431,#11433,#11434))
REPRESENTATION_CONTEXT('','3D')
);
#11431=(
LENGTH_UNIT()
NAMED_UNIT(*)
SI_UNIT(.MILLI.,.METRE.)
);
#11433=(
NAMED_UNIT(*)
PLANE_ANGLE_UNIT()
SI_UNIT($,.RADIAN.)
);
#11434=(
NAMED_UNIT(*)
SI_UNIT($,.STERADIAN.)
SOLID_ANGLE_UNIT()
);
#11440=SHAPE_DEFINITION_REPRESENTATION(#11453,#11483);
#11453=PRODUCT_DEFINITION_SHAPE('',$,#11497);
#11483=SHAPE_REPRESENTATION('',(#4742),#11422);
#11491=PRODUCT_DEFINITION_CONTEXT('part definition',#11532,'design');
#11497=PRODUCT_DEFINITION('2026-10-25-00-55-37-930',
'05_Pitch_Yoke_Gold_Anodised',#11510,#11491);
#11510=PRODUCT_DEFINITION_FORMATION('',$,#11539);
#11532=APPLICATION_CONTEXT(
'Core Data for Automotive Mechanical Design Process');
#11533=PRODUCT_CONTEXT('part definition',#11532,'mechanical');
#11539=PRODUCT('2026-10-25-00-55-37-930','05_Pitch_Yoke_Gold_Anodised',
$,(#11533));
#11617=COLOUR_RGB('Off White',0.89,0.88,0.83);
#11618=FILL_AREA_STYLE_COLOUR('',#11617);
#11619=FILL_AREA_STYLE('',(#11618));
#11620=SURFACE_STYLE_FILL_AREA(#11619);
#11621=SURFACE_SIDE_STYLE('',(#11620));
#11622=SURFACE_STYLE_USAGE(.BOTH.,#11621);
#11623=PRESENTATION_STYLE_ASSIGNMENT((#11622));
ENDSEC;
END-ISO-10303-21;
